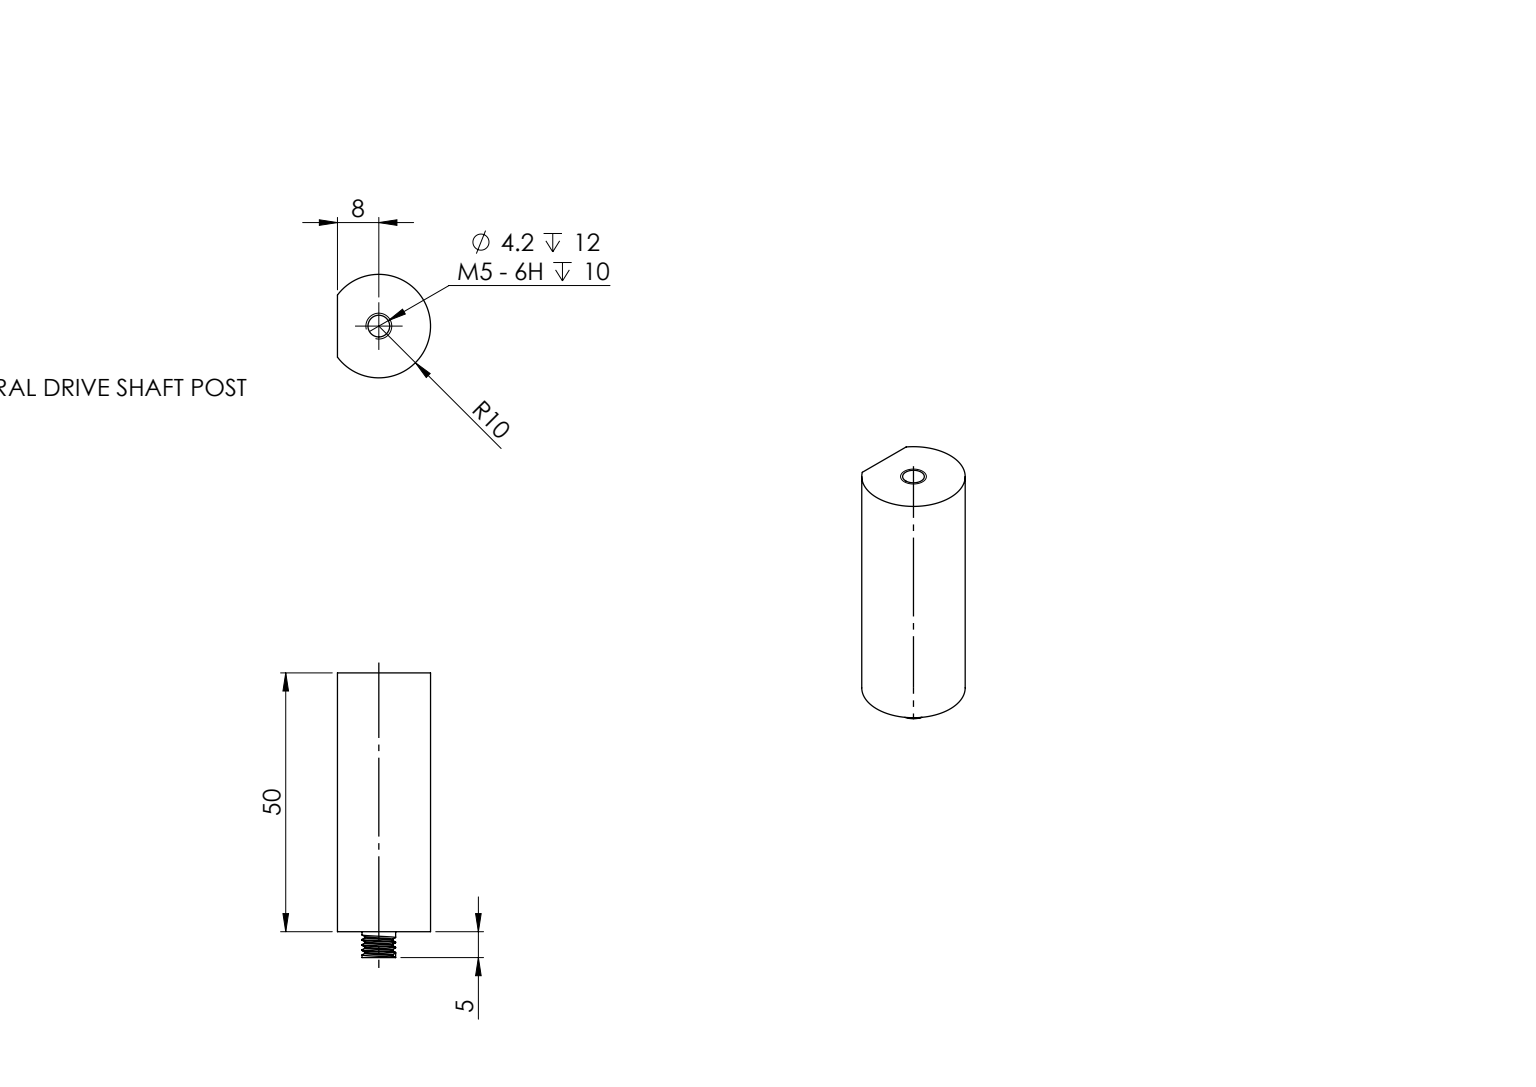
ISO-10303-21;
HEADER;
FILE_DESCRIPTION (('STEP AP214'),
    '1' );
FILE_NAME ('Central Drive Shaft Post.step',
    '2026-10-08T14:59:03',
    ( '' ),
    ( '' ),
    'SwSTEP 2.0',
    'SolidWorks 2026',
    '' );
FILE_SCHEMA (( 'AUTOMOTIVE_DESIGN' ));
ENDSEC;

DATA;
#13=CARTESIAN_POINT ( 'NONE',  ( -2.298097038856279806, 112.6250000000000000, -2.298097038856279362 ) ) ;
#14=CARTESIAN_POINT ( 'NONE',  ( 1.658621287961228320E-16, 111.8124999986344079, 2.708734124999999882 ) ) ;
#16=AXIS2_PLACEMENT_3D ( 'NONE', #8718, #1999, #3870 ) ;
#26=CARTESIAN_POINT ( 'NONE',  ( 0.000000000000000000, 153.0000000000000000, 2.099999999999998312 ) ) ;
#35=CARTESIAN_POINT ( 'NONE',  ( 3.250000000000000444, 113.0625000000000000, 1.346194077712559167 ) ) ;
#42=ORIENTED_EDGE ( 'NONE', *, *, #4224, .F. ) ;
#57=CARTESIAN_POINT ( 'NONE',  ( -1.915364268218909150, 112.6874999986344079, 1.915364268218909594 ) ) ;
#60=ORIENTED_EDGE ( 'NONE', *, *, #4267, .T. ) ;
#74=CARTESIAN_POINT ( 'NONE',  ( -3.250000000000000444, 111.5000000000000000, 3.980102097228898231E-16 ) ) ;
#90=ORIENTED_EDGE ( 'NONE', *, *, #4166, .T. ) ;
#101=CARTESIAN_POINT ( 'NONE',  ( -2.298097038856279362, 111.3750000000000000, 2.298097038856279806 ) ) ;
#103=CARTESIAN_POINT ( 'NONE',  ( 1.121994411437818862, 110.4999999986344079, 2.708734125000000326 ) ) ;
#122=CARTESIAN_POINT ( 'NONE',  ( -1.121994411437818862, 113.6249999986344079, 2.708734125000000326 ) ) ;
#124=EDGE_CURVE ( 'NONE', #2418, #8492, #10933, .T. ) ;
#126=EDGE_LOOP ( 'NONE', ( #8083, #10579, #5308 ) ) ;
#133=CARTESIAN_POINT ( 'NONE',  ( -1.346194077712560944, 110.3125000000000000, 3.249999999999998668 ) ) ;
#136=CARTESIAN_POINT ( 'NONE',  ( 1.915364268218908705, 114.4374999986344079, -1.915364268218909594 ) ) ;
#138=CARTESIAN_POINT ( 'NONE',  ( 1.915364268218909150, 112.6874999986344079, 1.915364268218909150 ) ) ;
#148=ADVANCED_FACE ( 'NONE', ( #9407 ), #4682, .T. ) ;
#153=EDGE_CURVE ( 'NONE', #12150, #6802, #1695, .T. ) ;
#167=CARTESIAN_POINT ( 'NONE',  ( 1.658621287961228566E-16, 110.5624999986344079, 2.708734125000000326 ) ) ;
#183=CARTESIAN_POINT ( 'NONE',  ( -2.708734125000000326, 113.7499999986343937, 1.121994411437818862 ) ) ;
#184=CARTESIAN_POINT ( 'NONE',  ( -5.970153145843347347E-16, 113.6249999972688158, -3.250000000000000444 ) ) ;
#196=EDGE_CURVE ( 'NONE', #8201, #12241, #11240, .T. ) ;
#217=AXIS2_PLACEMENT_3D ( 'NONE', #5378, #8352, #3567 ) ;
#232=CARTESIAN_POINT ( 'NONE',  ( 2.708734125000000326, 110.3749999986344221, 1.121994411437818862 ) ) ;
#239=CARTESIAN_POINT ( 'NONE',  ( -3.250000000000000444, 111.3124999972687874, 1.346194077712559167 ) ) ;
#245=ORIENTED_EDGE ( 'NONE', *, *, #2310, .T. ) ;
#246=CARTESIAN_POINT ( 'NONE',  ( -2.708734125000000326, 110.7499999986343937, 1.121994411437818862 ) ) ;
#249=EDGE_CURVE ( 'NONE', #1174, #5753, #3010, .T. ) ;
#263=CARTESIAN_POINT ( 'NONE',  ( -1.915364268218909594, 114.1874999986344079, -1.915364268218908927 ) ) ;
#265=CARTESIAN_POINT ( 'NONE',  ( -1.915364268218909594, 113.1874999986344079, -1.915364268218908927 ) ) ;
#289=CARTESIAN_POINT ( 'NONE',  ( -1.121994411437820416, 110.9999999986343937, -2.708734124999999882 ) ) ;
#291=CARTESIAN_POINT ( 'NONE',  ( 1.990051048614449116E-16, 113.1249999972688158, 3.250000000000000444 ) ) ;
#292=( GEOMETRIC_REPRESENTATION_CONTEXT ( 3 ) GLOBAL_UNCERTAINTY_ASSIGNED_CONTEXT ( ( #10000 ) ) GLOBAL_UNIT_ASSIGNED_CONTEXT ( ( #7020, #9690, #6089 ) ) REPRESENTATION_CONTEXT ( 'NONE', 'WORKASPACE' ) );
#307=CLOSED_SHELL ( 'NONE', ( #11275, #6512, #7917, #11356, #3953, #6283, #1808, #1279, #6245, #3383, #11433, #6682, #11026, #12101, #4967, #2002, #12145, #10844, #5599, #3792, #148, #6574, #11472, #11341, #11642, #320 ) ) ;
#308=CARTESIAN_POINT ( 'NONE',  ( -4.975863863883684959E-16, 111.0624999986344079, -2.708734125000000326 ) ) ;
#310=CARTESIAN_POINT ( 'NONE',  ( -2.298097038856279362, 114.2499999972688158, 2.298097038856279806 ) ) ;
#320=ADVANCED_FACE ( 'NONE', ( #4060 ), #2414, .F. ) ;
#324=ORIENTED_EDGE ( 'NONE', *, *, #11720, .F. ) ;
#325=CARTESIAN_POINT ( 'NONE',  ( -8.000000000000000000, 115.0000000000000000, 5.999999999999998224 ) ) ;
#337=VECTOR ( 'NONE', #4948, 1000.000000000000227 ) ;
#340=CARTESIAN_POINT ( 'NONE',  ( 1.121994411437819084, 110.4999999986343937, 2.708734125000000326 ) ) ;
#341=ORIENTED_EDGE ( 'NONE', *, *, #9592, .T. ) ;
#348=EDGE_CURVE ( 'NONE', #9835, #9973, #11157, .T. ) ;
#350=CARTESIAN_POINT ( 'NONE',  ( 2.708734124999999882, 114.2499999986344079, -1.121994411437820638 ) ) ;
#359=ORIENTED_EDGE ( 'NONE', *, *, #2691, .F. ) ;
#360=CARTESIAN_POINT ( 'NONE',  ( 0.000000000000000000, 165.0000000000000000, 0.000000000000000000 ) ) ;
#363=CARTESIAN_POINT ( 'NONE',  ( 0.000000000000000000, 165.0000000000000000, 0.000000000000000000 ) ) ;
#398=CARTESIAN_POINT ( 'NONE',  ( -3.250000000000000444, 112.3124999972687874, 1.346194077712559167 ) ) ;
#403=ORIENTED_EDGE ( 'NONE', *, *, #1223, .T. ) ;
#416=CARTESIAN_POINT ( 'NONE',  ( -2.708734125000000326, 113.8124999986344079, 3.317242575922457132E-16 ) ) ;
#418=FACE_OUTER_BOUND ( 'NONE', #10833, .T. ) ;
#421=VERTEX_POINT ( 'NONE', #5825 ) ;
#438=ORIENTED_EDGE ( 'NONE', *, *, #2215, .F. ) ;
#454=CARTESIAN_POINT ( 'NONE',  ( 3.250000000000000444, 111.0000000000000000, 0.000000000000000000 ) ) ;
#478=CARTESIAN_POINT ( 'NONE',  ( -4.975863863883684959E-16, 114.0624999986344079, -2.708734125000000326 ) ) ;
#480=CYLINDRICAL_SURFACE ( 'NONE', #7570, 3.250000000000000444 ) ;
#489=CARTESIAN_POINT ( 'NONE',  ( 2.298097038856279806, 113.9999999972688158, 2.298097038856279806 ) ) ;
#494=ORIENTED_EDGE ( 'NONE', *, *, #4807, .F. ) ;
#499=CARTESIAN_POINT ( 'NONE',  ( 1.990051048614449116E-16, 114.1249999972688158, 3.250000000000000444 ) ) ;
#509=CARTESIAN_POINT ( 'NONE',  ( 2.298097038856279806, 112.1250000000000000, 2.298097038856279806 ) ) ;
#525=CARTESIAN_POINT ( 'NONE',  ( 2.708734124999999882, 112.2499999986343937, -1.121994411437820416 ) ) ;
#529=ORIENTED_EDGE ( 'NONE', *, *, #10124, .T. ) ;
#540=CARTESIAN_POINT ( 'NONE',  ( 1.121994411437819528, 114.1249999986344079, -2.708734124999999882 ) ) ;
#541=CARTESIAN_POINT ( 'NONE',  ( -1.121994411437819084, 110.8749999986343937, 2.708734124999999882 ) ) ;
#551=ORIENTED_EDGE ( 'NONE', *, *, #4637, .F. ) ;
#586=CARTESIAN_POINT ( 'NONE',  ( 1.915364268218908927, 113.1874999986344079, -1.915364268218909816 ) ) ;
#589=MANIFOLD_SOLID_BREP ( 'Thread1', #307 ) ;
#605=CARTESIAN_POINT ( 'NONE',  ( 1.346194077712559389, 113.1875000000000142, 3.250000000000000444 ) ) ;
#618=EDGE_LOOP ( 'NONE', ( #8709, #551, #5002, #341 ) ) ;
#622=DIRECTION ( 'NONE',  ( -0.000000000000000000, 1.000000000000000000, -0.000000000000000000 ) ) ;
#627=CARTESIAN_POINT ( 'NONE',  ( -3.250000000000000444, 114.3749999972688158, 3.980102097228898231E-16 ) ) ;
#637=CARTESIAN_POINT ( 'NONE',  ( 2.298097038856278918, 111.8750000000000000, -2.298097038856279806 ) ) ;
#653=CARTESIAN_POINT ( 'NONE',  ( 1.121994411437819528, 114.1249999986344079, -2.708734124999999882 ) ) ;
#655=CARTESIAN_POINT ( 'NONE',  ( 1.121994411437818862, 111.7499999986344079, 2.708734124999999882 ) ) ;
#663=LINE ( 'NONE', #3470, #9246 ) ;
#665=DIRECTION ( 'NONE',  ( -0.000000000000000000, -1.000000000000000000, -0.000000000000000000 ) ) ;
#668=CARTESIAN_POINT ( 'NONE',  ( -5.970153145843347347E-16, 112.7500000000000000, -3.250000000000000444 ) ) ;
#685=AXIS2_PLACEMENT_3D ( 'NONE', #9077, #3726, #10139 ) ;
#704=CARTESIAN_POINT ( 'NONE',  ( 0.000000000000000000, 110.0000000000000000, 0.000000000000000000 ) ) ;
#705=MECHANICAL_DESIGN_GEOMETRIC_PRESENTATION_REPRESENTATION('',(#6077),#292);
#707=VECTOR ( 'NONE', #7770, 1000.000000000000000 ) ;
#709=EDGE_LOOP ( 'NONE', ( #12315, #3463 ) ) ;
#723=CARTESIAN_POINT ( 'NONE',  ( -2.708734124999999882, 110.9999999986343937, 1.121994411437818862 ) ) ;
#725=AXIS2_PLACEMENT_3D ( 'NONE', #3282, #2404, #5224 ) ;
#738=CARTESIAN_POINT ( 'NONE',  ( 3.250000000000000444, 113.0000000000000000, 0.000000000000000000 ) ) ;
#769=CARTESIAN_POINT ( 'NONE',  ( 2.708734124999999437, 114.4999999986344079, -1.121994411437820638 ) ) ;
#772=ORIENTED_EDGE ( 'NONE', *, *, #7001, .F. ) ;
#782=ORIENTED_EDGE ( 'NONE', *, *, #11976, .F. ) ;
#785=CARTESIAN_POINT ( 'NONE',  ( 1.915364268218908705, 113.4374999986344079, -1.915364268218909594 ) ) ;
#796=CARTESIAN_POINT ( 'NONE',  ( 2.298097038856279806, 112.1250000000000000, 2.298097038856279806 ) ) ;
#804=LINE ( 'NONE', #2726, #2890 ) ;
#829=CARTESIAN_POINT ( 'NONE',  ( 2.708734124999999882, 114.5624999986344079, 0.000000000000000000 ) ) ;
#843=CARTESIAN_POINT ( 'NONE',  ( -4.975863863883684959E-16, 113.3124999986344079, -2.708734124999999882 ) ) ;
#850=AXIS2_PLACEMENT_3D ( 'NONE', #3146, #7011, #2387 ) ;
#859=CARTESIAN_POINT ( 'NONE',  ( 2.298097038856278918, 112.7499999972688158, -2.298097038856279806 ) ) ;
#861=VERTEX_POINT ( 'NONE', #10306 ) ;
#887=CARTESIAN_POINT ( 'NONE',  ( 1.121994411437818862, 112.7499999986343937, 2.708734124999999882 ) ) ;
#889=CARTESIAN_POINT ( 'NONE',  ( 2.298097038856278918, 113.8750000000000000, -2.298097038856279806 ) ) ;
#902=CARTESIAN_POINT ( 'NONE',  ( 2.708734124999999882, 111.5624999986344079, 0.000000000000000000 ) ) ;
#917=CARTESIAN_POINT ( 'NONE',  ( -5.970153145843347347E-16, 112.7500000000000000, -3.250000000000000444 ) ) ;
#947=DIRECTION ( 'NONE',  ( 0.000000000000000000, 0.000000000000000000, -1.000000000000000000 ) ) ;
#951=CARTESIAN_POINT ( 'NONE',  ( 2.708734124999999882, 112.5624999986344079, 0.000000000000000000 ) ) ;
#952=CARTESIAN_POINT ( 'NONE',  ( -2.298097038856279362, 111.2499999972688158, 2.298097038856279806 ) ) ;
#965=CARTESIAN_POINT ( 'NONE',  ( -2.708734124999999882, 114.0624999986344079, 3.317242575922456639E-16 ) ) ;
#977=LINE ( 'NONE', #3904, #10328 ) ;
#995=CARTESIAN_POINT ( 'NONE',  ( -3.250000000000000444, 113.3124999972687874, 1.346194077712559167 ) ) ;
#1010=CARTESIAN_POINT ( 'NONE',  ( -2.708734125000000326, 113.1249999986343937, -1.121994411437818195 ) ) ;
#1011=CARTESIAN_POINT ( 'NONE',  ( -3.250000000000000444, 112.3749999972688158, 3.980102097228898231E-16 ) ) ;
#1025=DIRECTION ( 'NONE',  ( 0.000000000000000000, 0.000000000000000000, 1.000000000000000000 ) ) ;
#1026=CARTESIAN_POINT ( 'NONE',  ( -3.250000000000001776, 113.5625000000000000, -1.346194077712558723 ) ) ;
#1039=( LENGTH_UNIT ( ) NAMED_UNIT ( * ) SI_UNIT ( .MILLI., .METRE. ) );
#1041=APPLICATION_CONTEXT ( 'automotive_design' ) ;
#1053=CARTESIAN_POINT ( 'NONE',  ( -2.298097038856279362, 113.2499999972688158, 2.298097038856279806 ) ) ;
#1056=LINE ( 'NONE', #1122, #1359 ) ;
#1068=CARTESIAN_POINT ( 'NONE',  ( 1.915364268218908927, 113.1874999986344079, -1.915364268218909816 ) ) ;
#1070=CARTESIAN_POINT ( 'NONE',  ( -3.250000000000001776, 113.4374999972688300, -1.346194077712558723 ) ) ;
#1076=CARTESIAN_POINT ( 'NONE',  ( 0.000000000000000000, 165.0000000000000000, 0.000000000000000000 ) ) ;
#1099=CARTESIAN_POINT ( 'NONE',  ( -1.915364268218909150, 110.6874999986344079, 1.915364268218909594 ) ) ;
#1115=CARTESIAN_POINT ( 'NONE',  ( -2.708734125000000326, 110.8124999986344079, 3.317242575922457132E-16 ) ) ;
#1122=CARTESIAN_POINT ( 'NONE',  ( 2.571758278209433575E-16, 165.0000000000000000, -2.099999999999993427 ) ) ;
#1133=CARTESIAN_POINT ( 'NONE',  ( -1.915364268218909816, 113.9374999986344079, -1.915364268218909150 ) ) ;
#1134=CARTESIAN_POINT ( 'NONE',  ( -1.346194077712560944, 112.5624999972688158, -3.249999999999999556 ) ) ;
#1149=PLANE ( 'NONE',  #1794 ) ;
#1152=EDGE_CURVE ( 'NONE', #5494, #3256, #5047, .T. ) ;
#1153=VERTEX_POINT ( 'NONE', #9045 ) ;
#1160=CARTESIAN_POINT ( 'NONE',  ( 2.708734125000000326, 111.3124999986344079, 0.000000000000000000 ) ) ;
#1168=CARTESIAN_POINT ( 'NONE',  ( -2.708734125000000326, 112.1249999986343937, -1.121994411437818195 ) ) ;
#1174=VERTEX_POINT ( 'NONE', #4317 ) ;
#1185=ORIENTED_EDGE ( 'NONE', *, *, #4989, .T. ) ;
#1189=PRODUCT_CONTEXT ( 'NONE', #1041, 'mechanical' ) ;
#1194=CARTESIAN_POINT ( 'NONE',  ( 2.708734125000000326, 111.3124999986344079, 0.000000000000000000 ) ) ;
#1195=CARTESIAN_POINT ( 'NONE',  ( -3.250000000000000444, 111.3749999972688158, 3.980102097228898231E-16 ) ) ;
#1210=CARTESIAN_POINT ( 'NONE',  ( 1.121994411437819084, 112.3749999986344079, -2.708734124999999437 ) ) ;
#1223=EDGE_CURVE ( 'NONE', #9534, #3450, #11896, .T. ) ;
#1229=CARTESIAN_POINT ( 'NONE',  ( 3.980102097228898231E-16, 110.0000000000000000, -3.250000000000000444 ) ) ;
#1235=CARTESIAN_POINT ( 'NONE',  ( 2.708734125000000326, 112.3749999986344221, 1.121994411437818862 ) ) ;
#1239=( BOUNDED_CURVE ( )  B_SPLINE_CURVE ( 2, ( #499, #8154, #2434, #10086, #627, #11860, #10030, #5367, #11982 ),
 .UNSPECIFIED., .F., .F. ) 
 B_SPLINE_CURVE_WITH_KNOTS ( ( 3, 2, 2, 2, 3 ),
 ( 0.8125000000000006661, 0.8437500000000006661, 0.8750000000000006661, 0.9062500000000007772, 0.9375000000000007772 ),
 .UNSPECIFIED. ) 
 CURVE ( )  GEOMETRIC_REPRESENTATION_ITEM ( )  RATIONAL_B_SPLINE_CURVE ( ( 0.9999999999999983347, 0.9238795325112884038, 1.000000000000000000, 0.9238795325112867385, 1.000000000000000000, 0.9238795325112867385, 1.000000000000000000, 0.9238795325112848511, 1.000000000000001998 ) ) 
 REPRESENTATION_ITEM ( '' )  );
#1252=CARTESIAN_POINT ( 'NONE',  ( 2.708734124999999882, 111.2499999986344079, -1.121994411437820638 ) ) ;
#1253=CARTESIAN_POINT ( 'NONE',  ( 3.249999999999999556, 113.8124999972688016, -1.346194077712561610 ) ) ;
#1256=EDGE_CURVE ( 'NONE', #1921, #9884, #2097, .T. ) ;
#1263=CARTESIAN_POINT ( 'NONE',  ( -2.298097038856279362, 110.3750000000000000, 2.298097038856279806 ) ) ;
#1267=ORIENTED_EDGE ( 'NONE', *, *, #6550, .T. ) ;
#1274=ORIENTED_EDGE ( 'NONE', *, *, #3107, .T. ) ;
#1277=CARTESIAN_POINT ( 'NONE',  ( 1.990051048614449116E-16, 110.2500000000000000, 3.250000000000000444 ) ) ;
#1279=ADVANCED_FACE ( 'NONE', ( #5699 ), #5517, .T. ) ;
#1295=CARTESIAN_POINT ( 'NONE',  ( -1.915364268218909150, 111.6874999986344079, 1.915364268218909594 ) ) ;
#1314=CARTESIAN_POINT ( 'NONE',  ( -1.915364268218909150, 111.6874999986344079, 1.915364268218909594 ) ) ;
#1323=CARTESIAN_POINT ( 'NONE',  ( 0.000000000000000000, 110.0000000000000000, 0.000000000000000000 ) ) ;
#1347=SURFACE_SIDE_STYLE ('',( #4211 ) ) ;
#1355=CARTESIAN_POINT ( 'NONE',  ( -2.708734125000000326, 111.7499999986344079, 1.121994411437818862 ) ) ;
#1357=CARTESIAN_POINT ( 'NONE',  ( 0.000000000000000000, 165.0000000000000000, 0.000000000000000000 ) ) ;
#1359=VECTOR ( 'NONE', #1537, 1000.000000000000000 ) ;
#1377=EDGE_CURVE ( 'NONE', #8030, #8106, #3017, .T. ) ;
#1395=CARTESIAN_POINT ( 'NONE',  ( 3.249999999999999556, 110.9375000000000000, -1.346194077712561166 ) ) ;
#1417=CARTESIAN_POINT ( 'NONE',  ( 0.000000000000000000, 165.0000000000000000, -9.999999999999998224 ) ) ;
#1419=CARTESIAN_POINT ( 'NONE',  ( -1.915364268218909150, 113.6874999986344079, 1.915364268218909594 ) ) ;
#1459=CARTESIAN_POINT ( 'NONE',  ( 1.990051048614449116E-16, 111.2500000000000000, 3.250000000000000444 ) ) ;
#1462=ORIENTED_EDGE ( 'NONE', *, *, #11573, .T. ) ;
#1463=CARTESIAN_POINT ( 'NONE',  ( 1.990051048614449116E-16, 113.1249999972688158, 3.250000000000000444 ) ) ;
#1466=CARTESIAN_POINT ( 'NONE',  ( -1.915364268218909150, 112.6874999986344079, 1.915364268218909594 ) ) ;
#1476=DIRECTION ( 'NONE',  ( 0.000000000000000000, 0.000000000000000000, 1.000000000000000000 ) ) ;
#1481=CARTESIAN_POINT ( 'NONE',  ( 2.708734124999999882, 113.2499999986344079, -1.121994411437820638 ) ) ;
#1497=AXIS2_PLACEMENT_3D ( 'NONE', #7319, #7066, #11118 ) ;
#1502=PLANE ( 'NONE',  #9393 ) ;
#1520=DIRECTION ( 'NONE',  ( 0.000000000000000000, 0.000000000000000000, 1.000000000000000000 ) ) ;
#1528=CARTESIAN_POINT ( 'NONE',  ( -1.915364268218909816, 111.9374999986344079, -1.915364268218909150 ) ) ;
#1532=( LENGTH_UNIT ( ) NAMED_UNIT ( * ) SI_UNIT ( .MILLI., .METRE. ) );
#1534=UNCERTAINTY_MEASURE_WITH_UNIT (LENGTH_MEASURE( 1.000000000000000082E-05 ), #1039, 'distance_accuracy_value', 'NONE');
#1537=DIRECTION ( 'NONE',  ( -0.000000000000000000, 1.000000000000000000, -0.000000000000000000 ) ) ;
#1544=CARTESIAN_POINT ( 'NONE',  ( -2.298097038856279362, 112.3750000000000000, 2.298097038856279806 ) ) ;
#1545=CARTESIAN_POINT ( 'NONE',  ( 2.708734124999999882, 110.6249999986343937, 1.121994411437819084 ) ) ;
#1547=CARTESIAN_POINT ( 'NONE',  ( 3.249999999999999556, 112.8124999972687874, -1.346194077712561166 ) ) ;
#1550=VERTEX_POINT ( 'NONE', #9028 ) ;
#1561=VECTOR ( 'NONE', #11409, 1000.000000000000000 ) ;
#1568=AXIS2_PLACEMENT_3D ( 'NONE', #1776, #5529, #7332 ) ;
#1575=CARTESIAN_POINT ( 'NONE',  ( -5.970153145843347347E-16, 111.7500000000000000, -3.250000000000000444 ) ) ;
#1587=CARTESIAN_POINT ( 'NONE',  ( 1.915364268218909594, 112.4374999986344079, 1.915364268218909594 ) ) ;
#1590=CARTESIAN_POINT ( 'NONE',  ( -2.708734124999999882, 112.0624999986344079, 3.317242575922456639E-16 ) ) ;
#1603=CARTESIAN_POINT ( 'NONE',  ( 2.298097038856278918, 111.7499999972688158, -2.298097038856279806 ) ) ;
#1604=CARTESIAN_POINT ( 'NONE',  ( -2.298097038856279806, 111.6250000000000000, -2.298097038856279362 ) ) ;
#1612=AXIS2_PLACEMENT_3D ( 'NONE', #9562, #7823, #5032 ) ;
#1627=FACE_OUTER_BOUND ( 'NONE', #4261, .T. ) ;
#1640=EDGE_LOOP ( 'NONE', ( #4892, #782, #4872, #2457 ) ) ;
#1641=CARTESIAN_POINT ( 'NONE',  ( 2.708734124999999882, 110.5624999986344079, 0.000000000000000000 ) ) ;
#1652=CARTESIAN_POINT ( 'NONE',  ( -1.121994411437820194, 111.2499999986344079, -2.708734124999999437 ) ) ;
#1664=CARTESIAN_POINT ( 'NONE',  ( 1.346194077712559833, 112.8124999999999858, -3.250000000000000000 ) ) ;
#1676=EDGE_LOOP ( 'NONE', ( #6465, #3810, #10461, #7615 ) ) ;
#1686=DIRECTION ( 'NONE',  ( -0.000000000000000000, 1.000000000000000000, -0.000000000000000000 ) ) ;
#1695=( BOUNDED_CURVE ( )  B_SPLINE_CURVE ( 2, ( #2630, #1701, #889, #7437, #8474 ),
 .UNSPECIFIED., .F., .F. ) 
 B_SPLINE_CURVE_WITH_KNOTS ( ( 3, 2, 3 ),
 ( 0.9375000000000007772, 0.9687500000000004441, 1.000000000000000000 ),
 .UNSPECIFIED. ) 
 CURVE ( )  GEOMETRIC_REPRESENTATION_ITEM ( )  RATIONAL_B_SPLINE_CURVE ( ( 0.9999999999999981126, 0.9238795325112886259, 1.000000000000000000, 0.9238795325112867385, 1.000000000000000000 ) ) 
 REPRESENTATION_ITEM ( '' )  );
#1700=CARTESIAN_POINT ( 'NONE',  ( -1.121994411437818862, 112.8749999986344079, 2.708734124999999882 ) ) ;
#1701=CARTESIAN_POINT ( 'NONE',  ( 1.346194077712585591, 113.8125000000000142, -3.249999999999974687 ) ) ;
#1704=ORIENTED_EDGE ( 'NONE', *, *, #10723, .F. ) ;
#1715=CARTESIAN_POINT ( 'NONE',  ( -2.708734124999999882, 113.0624999986344079, 3.317242575922456639E-16 ) ) ;
#1722=CYLINDRICAL_SURFACE ( 'NONE', #1568, 3.250000000000000444 ) ;
#1730=CARTESIAN_POINT ( 'NONE',  ( -3.250000000000001776, 111.5624999999999858, -1.346194077712558723 ) ) ;
#1733=CARTESIAN_POINT ( 'NONE',  ( 1.990051048614449116E-16, 113.1249999972688158, 3.250000000000000444 ) ) ;
#1754=LINE ( 'NONE', #5438, #2930 ) ;
#1758=CARTESIAN_POINT ( 'NONE',  ( 1.658621287961228320E-16, 113.8124999986344079, 2.708734124999999882 ) ) ;
#1764=ORIENTED_EDGE ( 'NONE', *, *, #124, .F. ) ;
#1770=CARTESIAN_POINT ( 'NONE',  ( 1.658621287961228320E-16, 111.8124999986344079, 2.708734124999999882 ) ) ;
#1771=CARTESIAN_POINT ( 'NONE',  ( -1.121994411437820194, 111.2499999986344079, -2.708734124999999437 ) ) ;
#1776=CARTESIAN_POINT ( 'NONE',  ( 0.000000000000000000, 110.0000000000000000, 0.000000000000000000 ) ) ;
#1794=AXIS2_PLACEMENT_3D ( 'NONE', #6754, #11627, #4951 ) ;
#1806=LINE ( 'NONE', #11225, #8415 ) ;
#1808=ADVANCED_FACE ( 'NONE', ( #2163 ), #10942, .T. ) ;
#1813=CARTESIAN_POINT ( 'NONE',  ( 3.250000000000000444, 110.0000000000000000, 0.000000000000000000 ) ) ;
#1814=VECTOR ( 'NONE', #6503, 1000.000000000000000 ) ;
#1817=CARTESIAN_POINT ( 'NONE',  ( -4.975863863883684959E-16, 112.3124999986344079, -2.708734124999999882 ) ) ;
#1826=CARTESIAN_POINT ( 'NONE',  ( 3.250000000000000444, 110.0624999999999858, 1.346194077712559167 ) ) ;
#1832=CARTESIAN_POINT ( 'NONE',  ( 1.915364268218909150, 110.6874999986344079, 1.915364268218909150 ) ) ;
#1874=CARTESIAN_POINT ( 'NONE',  ( 1.915364268218908705, 114.4374999986344079, -1.915364268218909594 ) ) ;
#1876=CARTESIAN_POINT ( 'NONE',  ( -2.298097038856279806, 111.4999999972688158, -2.298097038856279362 ) ) ;
#1883=CARTESIAN_POINT ( 'NONE',  ( -5.970153145843347347E-16, 112.7500000000000000, -3.250000000000000444 ) ) ;
#1921=VERTEX_POINT ( 'NONE', #11007 ) ;
#1927=ORIENTED_EDGE ( 'NONE', *, *, #4103, .F. ) ;
#1933=CARTESIAN_POINT ( 'NONE',  ( -5.970153145843347347E-16, 111.6249999972688158, -3.250000000000000444 ) ) ;
#1942=CARTESIAN_POINT ( 'NONE',  ( 1.658621287961228320E-16, 112.8124999986344079, 2.708734124999999882 ) ) ;
#1943=CARTESIAN_POINT ( 'NONE',  ( 1.346194077712559389, 111.0624999972688016, 3.250000000000000444 ) ) ;
#1948=CARTESIAN_POINT ( 'NONE',  ( 2.298097038856279806, 110.1250000000000000, 2.298097038856279806 ) ) ;
#1953=CARTESIAN_POINT ( 'NONE',  ( -1.121994411437820194, 114.2499999986344079, -2.708734124999999437 ) ) ;
#1954=CARTESIAN_POINT ( 'NONE',  ( 2.298097038856278918, 113.8750000000000000, -2.298097038856279806 ) ) ;
#1959=MECHANICAL_DESIGN_GEOMETRIC_PRESENTATION_REPRESENTATION('',(#10160),#3359);
#1999=DIRECTION ( 'NONE',  ( 0.000000000000000000, 1.000000000000000000, 0.000000000000000000 ) ) ;
#2001=CARTESIAN_POINT ( 'NONE',  ( -2.708734125000000326, 112.8124999986344079, 3.317242575922457132E-16 ) ) ;
#2002=ADVANCED_FACE ( 'NONE', ( #3469 ), #11075, .F. ) ;
#2003=CARTESIAN_POINT ( 'NONE',  ( 2.298097038856278918, 111.7499999972688158, -2.298097038856279806 ) ) ;
#2018=CARTESIAN_POINT ( 'NONE',  ( 0.000000000000000000, 165.0000000000000000, 0.000000000000000000 ) ) ;
#2021=CARTESIAN_POINT ( 'NONE',  ( 1.915364268218909150, 113.6874999986344079, 1.915364268218909150 ) ) ;
#2029=AXIS2_PLACEMENT_3D ( 'NONE', #4331, #8256, #6334 ) ;
#2034=CARTESIAN_POINT ( 'NONE',  ( -1.915364268218909816, 110.9374999986344079, -1.915364268218909150 ) ) ;
#2066=CARTESIAN_POINT ( 'NONE',  ( 1.346194077712559833, 112.6874999972688158, -3.250000000000000000 ) ) ;
#2079=CARTESIAN_POINT ( 'NONE',  ( 1.121994411437819084, 114.3749999986344221, -2.708734124999999437 ) ) ;
#2081=CARTESIAN_POINT ( 'NONE',  ( 2.708734124999999437, 114.4999999986344079, -1.121994411437820416 ) ) ;
#2093=CARTESIAN_POINT ( 'NONE',  ( -2.708734125000000326, 110.7499999986343937, 1.121994411437819084 ) ) ;
#2097=( BOUNDED_CURVE ( )  B_SPLINE_CURVE ( 2, ( #8481, #11182, #3753, #2636, #2697, #6444, #6509, #10235, #1883 ),
 .UNSPECIFIED., .F., .F. ) 
 B_SPLINE_CURVE_WITH_KNOTS ( ( 3, 2, 2, 2, 3 ),
 ( 0.5625000000000004441, 0.5937500000000004441, 0.6250000000000004441, 0.6562500000000005551, 0.6875000000000005551 ),
 .UNSPECIFIED. ) 
 CURVE ( )  GEOMETRIC_REPRESENTATION_ITEM ( )  RATIONAL_B_SPLINE_CURVE ( ( 0.9999999999999988898, 0.9238795325112878487, 1.000000000000000000, 0.9238795325112867385, 1.000000000000000000, 0.9238795325112867385, 1.000000000000000000, 0.9238795325112854062, 1.000000000000001332 ) ) 
 REPRESENTATION_ITEM ( '' )  );
#2103=FILL_AREA_STYLE ('',( #3219 ) ) ;
#2109=CARTESIAN_POINT ( 'NONE',  ( 1.990051048614449116E-16, 111.2500000000000000, 3.250000000000000444 ) ) ;
#2116=ORIENTED_EDGE ( 'NONE', *, *, #4989, .F. ) ;
#2125=FACE_BOUND ( 'NONE', #709, .T. ) ;
#2127=CARTESIAN_POINT ( 'NONE',  ( -1.915364268218909816, 111.9374999986344079, -1.915364268218909150 ) ) ;
#2128=CARTESIAN_POINT ( 'NONE',  ( -1.346194077712559389, 113.1874999972688016, 3.250000000000000444 ) ) ;
#2141=CARTESIAN_POINT ( 'NONE',  ( 0.000000000000000000, 153.0000000000000000, 0.000000000000000000 ) ) ;
#2143=CARTESIAN_POINT ( 'NONE',  ( 2.708734124999999437, 112.4999999986343937, -1.121994411437820416 ) ) ;
#2150=DIRECTION ( 'NONE',  ( 0.000000000000000000, 0.000000000000000000, 1.000000000000000000 ) ) ;
#2163=FACE_OUTER_BOUND ( 'NONE', #8054, .T. ) ;
#2179=CARTESIAN_POINT ( 'NONE',  ( -1.121994411437818862, 111.6249999986344079, 2.708734125000000326 ) ) ;
#2180=CARTESIAN_POINT ( 'NONE',  ( 1.990051048614449116E-16, 114.1249999972688158, 3.250000000000000444 ) ) ;
#2198=CARTESIAN_POINT ( 'NONE',  ( 2.708734124999999882, 111.6249999986343937, 1.121994411437819084 ) ) ;
#2209=CARTESIAN_POINT ( 'NONE',  ( 0.000000000000000000, 115.0000000000000000, -9.999999999999998224 ) ) ;
#2211=DIRECTION ( 'NONE',  ( 0.000000000000000000, 0.000000000000000000, -1.000000000000000000 ) ) ;
#2215=EDGE_CURVE ( 'NONE', #9788, #5829, #977, .T. ) ;
#2217=SURFACE_STYLE_USAGE ( .BOTH. , #1347 ) ;
#2220=SURFACE_SIDE_STYLE ('',( #11703 ) ) ;
#2221=AXIS2_PLACEMENT_3D ( 'NONE', #4678, #8469, #12295 ) ;
#2227=CARTESIAN_POINT ( 'NONE',  ( -4.975863863883684959E-16, 113.0624999986344079, -2.708734125000000326 ) ) ;
#2231=ORIENTED_EDGE ( 'NONE', *, *, #6662, .T. ) ;
#2241=CARTESIAN_POINT ( 'NONE',  ( -2.708734125000000770, 110.8749999986343937, -1.121994411437818639 ) ) ;
#2248=DIRECTION ( 'NONE',  ( -0.000000000000000000, 1.000000000000000000, -0.000000000000000000 ) ) ;
#2260=CARTESIAN_POINT ( 'NONE',  ( 1.990051048614449116E-16, 112.1249999972688158, 3.250000000000000444 ) ) ;
#2268=EDGE_LOOP ( 'NONE', ( #10266, #8033, #7306, #7027, #11755, #11420, #6855, #438 ) ) ;
#2271=CARTESIAN_POINT ( 'NONE',  ( 0.000000000000000000, 110.0000000000000000, 0.000000000000000000 ) ) ;
#2276=SHAPE_REPRESENTATION_RELATIONSHIP ( 'NONE' , 'NONE' ,  #7136, #7202 ) ;
#2278=ORIENTED_EDGE ( 'NONE', *, *, #9929, .T. ) ;
#2288=CARTESIAN_POINT ( 'NONE',  ( -3.250000000000000444, 110.4375000000000000, 1.346194077712559389 ) ) ;
#2310=EDGE_CURVE ( 'NONE', #2754, #4316, #4490, .T. ) ;
#2326=ORIENTED_EDGE ( 'NONE', *, *, #4166, .F. ) ;
#2333=CARTESIAN_POINT ( 'NONE',  ( 2.708734125000000326, 112.3749999986344079, 1.121994411437819084 ) ) ;
#2335=ORIENTED_EDGE ( 'NONE', *, *, #1377, .T. ) ;
#2346=CARTESIAN_POINT ( 'NONE',  ( -1.915364268218909816, 110.9374999986344079, -1.915364268218909150 ) ) ;
#2351=EDGE_CURVE ( 'NONE', #7682, #7936, #6187, .T. ) ;
#2362=CARTESIAN_POINT ( 'NONE',  ( 3.980102097228898231E-16, 110.0000000000000000, -3.250000000000000444 ) ) ;
#2377=CARTESIAN_POINT ( 'NONE',  ( 2.708734124999999882, 110.6249999986343937, 1.121994411437818862 ) ) ;
#2387=DIRECTION ( 'NONE',  ( 0.000000000000000000, 0.000000000000000000, -1.000000000000000000 ) ) ;
#2392=CARTESIAN_POINT ( 'NONE',  ( -1.121994411437820194, 112.9999999986344079, -2.708734124999999882 ) ) ;
#2404=DIRECTION ( 'NONE',  ( 0.000000000000000000, 1.000000000000000000, 0.000000000000000000 ) ) ;
#2408=CARTESIAN_POINT ( 'NONE',  ( -4.975863863883684959E-16, 111.0624999986344079, -2.708734125000000326 ) ) ;
#2414=( BOUNDED_SURFACE ( )  B_SPLINE_SURFACE ( 1, 2, ( 
 ( #2874, #4810, #6804, #1943, #7851, #9713, #952, #6679, #1195, #4996, #1876, #2941, #3938, #6741, #2003, #8661, #4745, #11613, #3062, #2813, #3997, #6866, #11548, #10600, #1011, #9654, #7736, #1134, #5810, #2066, #4936, #5751, #8723, #6617, #8533, #3812, #10661, #2128, #7613, #9596, #2999, #1070, #11422, #9531, #184, #8783, #6925, #1253, #5061, #5991, #3122, #9779, #2180, #10720, #310, #8841, #4119, #11670, #3698, #4449, #10240, #11316, #12310, #12252, #9237 ),
 ( #2582, #5523, #1832, #10365, #10301, #3641, #10110, #723, #5642, #7507, #6569, #1652, #11190, #6515, #9419, #2762, #902, #5458, #4693, #655, #1770, #3581, #9298, #6449, #1590, #8486, #2526, #6389, #11065, #5393, #9174, #7448, #12130, #11254, #7389, #3760, #8247, #2642, #8308, #5581, #1715, #6326, #12068, #3524, #843, #7327, #785, #11126, #4572, #4516, #8366, #10177, #12193, #2703, #9359, #4635, #8428, #5765, #263, #1953, #9609, #2079, #136, #9545, #3076 ) ),
 .UNSPECIFIED., .F., .F., .F. ) 
 B_SPLINE_SURFACE_WITH_KNOTS ( ( 2, 2 ),
 ( 3, 2, 2, 2, 2, 2, 2, 2, 2, 2, 2, 2, 2, 2, 2, 2, 2, 2, 2, 2, 2, 2, 2, 2, 2, 2, 2, 2, 2, 2, 2, 2, 3 ),
 ( 0.000000000000000000, 1.000000000000000000 ),
 ( 0.000000000000000000, 0.03125000000000000000, 0.06250000000000000000, 0.09375000000000000000, 0.1250000000000000000, 0.1562500000000000000, 0.1875000000000000000, 0.2187500000000000000, 0.2500000000000000000, 0.2812500000000000000, 0.3125000000000000000, 0.3437500000000000000, 0.3750000000000000000, 0.4062500000000000000, 0.4375000000000000000, 0.4687500000000000000, 0.5000000000000000000, 0.5312500000000000000, 0.5625000000000000000, 0.5937500000000000000, 0.6250000000000000000, 0.6562500000000000000, 0.6875000000000000000, 0.7187500000000000000, 0.7500000000000000000, 0.7812500000000000000, 0.8125000000000000000, 0.8437500000000000000, 0.8750000000000000000, 0.9062500000000000000, 0.9375000000000000000, 0.9687500000000000000, 1.000000000000000000 ),
 .UNSPECIFIED. ) 
 GEOMETRIC_REPRESENTATION_ITEM ( )  RATIONAL_B_SPLINE_SURFACE ( (
 ( 1.000000000000000000, 0.9238795325112867385, 1.000000000000000000, 0.9238795325112867385, 1.000000000000000000, 0.9238795325112867385, 1.000000000000000000, 0.9238795325112867385, 1.000000000000000000, 0.9238795325112867385, 1.000000000000000000, 0.9238795325112867385, 1.000000000000000000, 0.9238795325112867385, 1.000000000000000000, 0.9238795325112867385, 1.000000000000000000, 0.9238795325112867385, 1.000000000000000000, 0.9238795325112867385, 1.000000000000000000, 0.9238795325112867385, 1.000000000000000000, 0.9238795325112867385, 1.000000000000000000, 0.9238795325112867385, 1.000000000000000000, 0.9238795325112867385, 1.000000000000000000, 0.9238795325112867385, 1.000000000000000000, 0.9238795325112867385, 1.000000000000000000, 0.9238795325112867385, 1.000000000000000000, 0.9238795325112867385, 1.000000000000000000, 0.9238795325112867385, 1.000000000000000000, 0.9238795325112867385, 1.000000000000000000, 0.9238795325112867385, 1.000000000000000000, 0.9238795325112867385, 1.000000000000000000, 0.9238795325112867385, 1.000000000000000000, 0.9238795325112867385, 1.000000000000000000, 0.9238795325112867385, 1.000000000000000000, 0.9238795325112867385, 1.000000000000000000, 0.9238795325112867385, 1.000000000000000000, 0.9238795325112867385, 1.000000000000000000, 0.9238795325112867385, 1.000000000000000000, 0.9238795325112867385, 1.000000000000000000, 0.9238795325112867385, 1.000000000000000000, 0.9238795325112867385, 1.000000000000000000),
 ( 1.000000000000000000, 0.9238795325112867385, 1.000000000000000000, 0.9238795325112867385, 1.000000000000000000, 0.9238795325112867385, 1.000000000000000000, 0.9238795325112867385, 1.000000000000000000, 0.9238795325112867385, 1.000000000000000000, 0.9238795325112867385, 1.000000000000000000, 0.9238795325112867385, 1.000000000000000000, 0.9238795325112867385, 1.000000000000000000, 0.9238795325112867385, 1.000000000000000000, 0.9238795325112867385, 1.000000000000000000, 0.9238795325112867385, 1.000000000000000000, 0.9238795325112867385, 1.000000000000000000, 0.9238795325112867385, 1.000000000000000000, 0.9238795325112867385, 1.000000000000000000, 0.9238795325112867385, 1.000000000000000000, 0.9238795325112867385, 1.000000000000000000, 0.9238795325112867385, 1.000000000000000000, 0.9238795325112867385, 1.000000000000000000, 0.9238795325112867385, 1.000000000000000000, 0.9238795325112867385, 1.000000000000000000, 0.9238795325112867385, 1.000000000000000000, 0.9238795325112867385, 1.000000000000000000, 0.9238795325112867385, 1.000000000000000000, 0.9238795325112867385, 1.000000000000000000, 0.9238795325112867385, 1.000000000000000000, 0.9238795325112867385, 1.000000000000000000, 0.9238795325112867385, 1.000000000000000000, 0.9238795325112867385, 1.000000000000000000, 0.9238795325112867385, 1.000000000000000000, 0.9238795325112867385, 1.000000000000000000, 0.9238795325112867385, 1.000000000000000000, 0.9238795325112867385, 1.000000000000000000) ) ) 
 REPRESENTATION_ITEM ( '' )  SURFACE ( )  );
#2418=VERTEX_POINT ( 'NONE', #1641 ) ;
#2424=VECTOR ( 'NONE', #3740, 1000.000000000000000 ) ;
#2430=EDGE_CURVE ( 'NONE', #9973, #9835, #3998, .T. ) ;
#2434=CARTESIAN_POINT ( 'NONE',  ( -2.298097038856279362, 114.2499999972688158, 2.298097038856279806 ) ) ;
#2447=CARTESIAN_POINT ( 'NONE',  ( -1.121994411437818862, 110.8749999986343937, 2.708734124999999882 ) ) ;
#2457=ORIENTED_EDGE ( 'NONE', *, *, #11720, .T. ) ;
#2460=CARTESIAN_POINT ( 'NONE',  ( -4.975863863883684959E-16, 112.0624999986344079, -2.708734125000000326 ) ) ;
#2470=EDGE_CURVE ( 'NONE', #7137, #7682, #5448, .T. ) ;
#2478=CARTESIAN_POINT ( 'NONE',  ( 1.658621287961228566E-16, 113.5624999986344079, 2.708734125000000326 ) ) ;
#2479=CARTESIAN_POINT ( 'NONE',  ( -2.708734124999999882, 111.0624999986344079, 3.317242575922456639E-16 ) ) ;
#2525=CARTESIAN_POINT ( 'NONE',  ( -1.121994411437820194, 111.9999999986343937, -2.708734124999999882 ) ) ;
#2526=CARTESIAN_POINT ( 'NONE',  ( -1.915364268218909594, 112.1874999986344079, -1.915364268218908927 ) ) ;
#2539=CARTESIAN_POINT ( 'NONE',  ( 1.346194077712559833, 111.8125000000000000, -3.250000000000000000 ) ) ;
#2546=CARTESIAN_POINT ( 'NONE',  ( 1.346194077712537629, 114.0624999972688016, 3.250000000000022649 ) ) ;
#2548=APPLICATION_CONTEXT ( 'automotive_design' ) ;
#2552=VERTEX_POINT ( 'NONE', #12184 ) ;
#2561=PRODUCT_DEFINITION_FORMATION_WITH_SPECIFIED_SOURCE ( 'ANY', '', #8763, .NOT_KNOWN. ) ;
#2576=VERTEX_POINT ( 'NONE', #10540 ) ;
#2579=CARTESIAN_POINT ( 'NONE',  ( 2.708734125000000326, 114.3124999986344079, 0.000000000000000000 ) ) ;
#2582=CARTESIAN_POINT ( 'NONE',  ( 2.708734124999999882, 110.5624999986344079, 0.000000000000000000 ) ) ;
#2598=CARTESIAN_POINT ( 'NONE',  ( 1.346194077712559389, 111.1875000000000142, 3.250000000000000444 ) ) ;
#2600=CARTESIAN_POINT ( 'NONE',  ( 2.708734125000000326, 110.3124999986344079, 0.000000000000000000 ) ) ;
#2629=CARTESIAN_POINT ( 'NONE',  ( 1.915364268218908705, 111.4374999986344079, -1.915364268218909594 ) ) ;
#2630=CARTESIAN_POINT ( 'NONE',  ( -5.970153145843347347E-16, 113.7500000000000000, -3.250000000000000444 ) ) ;
#2636=CARTESIAN_POINT ( 'NONE',  ( -3.250000000000000444, 112.4375000000000000, 1.346194077712559167 ) ) ;
#2638=ORIENTED_EDGE ( 'NONE', *, *, #4576, .F. ) ;
#2642=CARTESIAN_POINT ( 'NONE',  ( -1.121994411437818862, 112.8749999986344079, 2.708734124999999882 ) ) ;
#2654=CARTESIAN_POINT ( 'NONE',  ( -3.250000000000001776, 112.5625000000000000, -1.346194077712558723 ) ) ;
#2687=CARTESIAN_POINT ( 'NONE',  ( 2.708734124999999882, 113.6249999986344079, 1.121994411437818862 ) ) ;
#2691=EDGE_CURVE ( 'NONE', #9973, #8106, #10416, .T. ) ;
#2697=CARTESIAN_POINT ( 'NONE',  ( -3.250000000000000444, 112.5000000000000000, 3.980102097228898231E-16 ) ) ;
#2703=CARTESIAN_POINT ( 'NONE',  ( -1.121994411437818862, 113.8749999986343937, 2.708734124999999882 ) ) ;
#2704=CARTESIAN_POINT ( 'NONE',  ( 2.708734124999999882, 111.5624999986344079, 0.000000000000000000 ) ) ;
#2715=LINE ( 'NONE', #3886, #9451 ) ;
#2720=AXIS2_PLACEMENT_3D ( 'NONE', #2271, #8057, #2211 ) ;
#2726=CARTESIAN_POINT ( 'NONE',  ( -8.000000000000000000, 165.0000000000000000, -5.999999999999998224 ) ) ;
#2738=VERTEX_POINT ( 'NONE', #7047 ) ;
#2748=CARTESIAN_POINT ( 'NONE',  ( -1.121994411437820194, 111.2499999986344079, -2.708734124999999437 ) ) ;
#2754=VERTEX_POINT ( 'NONE', #7170 ) ;
#2762=CARTESIAN_POINT ( 'NONE',  ( 2.708734124999999437, 111.4999999986343937, -1.121994411437820638 ) ) ;
#2784=CARTESIAN_POINT ( 'NONE',  ( 3.249999999999999556, 112.9375000000000000, -1.346194077712561166 ) ) ;
#2792=CARTESIAN_POINT ( 'NONE',  ( -8.000000000000000000, 165.0000000000000000, 5.999999999999998224 ) ) ;
#2812=CARTESIAN_POINT ( 'NONE',  ( -2.708734125000000326, 114.1249999986344079, -1.121994411437818195 ) ) ;
#2813=CARTESIAN_POINT ( 'NONE',  ( 1.346194077712559389, 112.0624999972688016, 3.250000000000000444 ) ) ;
#2822=CARTESIAN_POINT ( 'NONE',  ( 0.000000000000000000, 110.0000000000000000, 0.000000000000000000 ) ) ;
#2854=DIRECTION ( 'NONE',  ( -0.000000000000000000, 1.000000000000000000, -0.000000000000000000 ) ) ;
#2872=CARTESIAN_POINT ( 'NONE',  ( 2.708734124999999882, 112.6249999986343937, 1.121994411437818862 ) ) ;
#2874=CARTESIAN_POINT ( 'NONE',  ( 3.250000000000000444, 110.8749999972688158, 0.000000000000000000 ) ) ;
#2887=CARTESIAN_POINT ( 'NONE',  ( 1.990051048614449116E-16, 113.2500000000000000, 3.250000000000000444 ) ) ;
#2889=CARTESIAN_POINT ( 'NONE',  ( -2.708734125000000326, 114.1249999986344079, -1.121994411437818195 ) ) ;
#2890=VECTOR ( 'NONE', #7348, 1000.000000000000000 ) ;
#2913=( BOUNDED_CURVE ( )  B_SPLINE_CURVE ( 2, ( #8119, #6202, #9994, #4448, #8246 ),
 .UNSPECIFIED., .F., .F. ) 
 B_SPLINE_CURVE_WITH_KNOTS ( ( 3, 2, 3 ),
 ( 0.9375000000000007772, 0.9687500000000004441, 1.000000000000000000 ),
 .UNSPECIFIED. ) 
 CURVE ( )  GEOMETRIC_REPRESENTATION_ITEM ( )  RATIONAL_B_SPLINE_CURVE ( ( 0.9999999999999981126, 0.9238795325112886259, 1.000000000000000000, 0.9238795325112867385, 1.000000000000000000 ) ) 
 REPRESENTATION_ITEM ( '' )  );
#2922=CARTESIAN_POINT ( 'NONE',  ( 0.000000000000000000, 115.0000000000000000, 0.000000000000000000 ) ) ;
#2930=VECTOR ( 'NONE', #10980, 1000.000000000000000 ) ;
#2933=CARTESIAN_POINT ( 'NONE',  ( 0.000000000000000000, 165.0000000000000000, 2.099999999999988987 ) ) ;
#2940=CARTESIAN_POINT ( 'NONE',  ( 1.121994411437819528, 114.1249999986344079, -2.708734124999999882 ) ) ;
#2941=CARTESIAN_POINT ( 'NONE',  ( -1.346194077712560944, 111.5624999972688300, -3.249999999999999556 ) ) ;
#2954=CARTESIAN_POINT ( 'NONE',  ( 1.346194077712559833, 110.8124999999999858, -3.250000000000000000 ) ) ;
#2956=CARTESIAN_POINT ( 'NONE',  ( -2.708734124999999882, 111.9999999986343937, 1.121994411437819084 ) ) ;
#2981=CARTESIAN_POINT ( 'NONE',  ( 0.000000000000000000, 165.0000000000000000, 0.000000000000000000 ) ) ;
#2983=VECTOR ( 'NONE', #5875, 1000.000000000000000 ) ;
#2987=DIRECTION ( 'NONE',  ( 0.8660254037844408170, -0.4999999999999961697, 0.000000000000000000 ) ) ;
#2998=CARTESIAN_POINT ( 'NONE',  ( -4.975863863883684959E-16, 112.0624999986344079, -2.708734125000000326 ) ) ;
#2999=CARTESIAN_POINT ( 'NONE',  ( -3.250000000000000444, 113.3749999972688158, 3.980102097228898231E-16 ) ) ;
#3010=CIRCLE ( 'NONE', #7779, 3.250000000000000444 ) ;
#3017=CIRCLE ( 'NONE', #9773, 2.099999999999988987 ) ;
#3018=CARTESIAN_POINT ( 'NONE',  ( -1.915364268218909594, 112.1874999986344079, -1.915364268218908927 ) ) ;
#3037=CARTESIAN_POINT ( 'NONE',  ( 2.298097038856279806, 113.1250000000000000, 2.298097038856279806 ) ) ;
#3041=DIRECTION ( 'NONE',  ( 0.000000000000000000, -1.000000000000000000, 0.000000000000000000 ) ) ;
#3049=LINE ( 'NONE', #10467, #6934 ) ;
#3052=CARTESIAN_POINT ( 'NONE',  ( 0.000000000000000000, 110.0000000000000000, 0.000000000000000000 ) ) ;
#3055=SHAPE_DEFINITION_REPRESENTATION ( #6681, #7136 ) ;
#3057=EDGE_CURVE ( 'NONE', #12307, #9534, #3049, .T. ) ;
#3062=CARTESIAN_POINT ( 'NONE',  ( 2.298097038856279806, 111.9999999972688158, 2.298097038856279806 ) ) ;
#3076=CARTESIAN_POINT ( 'NONE',  ( 2.708734124999999882, 114.5624999986344079, 0.000000000000000000 ) ) ;
#3078=CARTESIAN_POINT ( 'NONE',  ( -1.915364268218908927, 113.9374999986344079, 1.915364268218909150 ) ) ;
#3079=CONICAL_SURFACE ( 'NONE', #685, 2.099999999999998312, 1.029744258676656532 ) ;
#3081=ORIENTED_EDGE ( 'NONE', *, *, #2310, .F. ) ;
#3107=EDGE_CURVE ( 'NONE', #2738, #8492, #3798, .T. ) ;
#3108=CIRCLE ( 'NONE', #725, 9.999999999999998224 ) ;
#3114=CARTESIAN_POINT ( 'NONE',  ( -5.970153145843347347E-16, 111.6249999972688158, -3.250000000000000444 ) ) ;
#3121=CARTESIAN_POINT ( 'NONE',  ( -1.121994411437820416, 111.9999999986343937, -2.708734124999999882 ) ) ;
#3122=CARTESIAN_POINT ( 'NONE',  ( 2.298097038856279806, 113.9999999972688158, 2.298097038856279806 ) ) ;
#3138=CARTESIAN_POINT ( 'NONE',  ( -1.121994411437820194, 114.2499999986344079, -2.708734124999999437 ) ) ;
#3146=CARTESIAN_POINT ( 'NONE',  ( 0.000000000000000000, 165.0000000000000000, 0.000000000000000000 ) ) ;
#3161=CARTESIAN_POINT ( 'NONE',  ( 1.658621287961228566E-16, 112.5624999986344079, 2.708734125000000326 ) ) ;
#3169=EDGE_CURVE ( 'NONE', #9835, #8030, #1056, .T. ) ;
#3179=CARTESIAN_POINT ( 'NONE',  ( 2.708734125000000326, 113.3749999986344079, 1.121994411437818862 ) ) ;
#3188=EDGE_LOOP ( 'NONE', ( #2326, #2231, #8721, #9253, #1704, #11944 ) ) ;
#3212=CARTESIAN_POINT ( 'NONE',  ( -1.121994411437819084, 110.6249999986343937, 2.708734125000000326 ) ) ;
#3215=PRESENTATION_STYLE_ASSIGNMENT (( #2217 ) ) ;
#3219=FILL_AREA_STYLE_COLOUR ( '', #11286 ) ;
#3228=CARTESIAN_POINT ( 'NONE',  ( -1.121994411437818862, 113.6249999986344079, 2.708734125000000326 ) ) ;
#3233=EDGE_LOOP ( 'NONE', ( #12284, #8659, #6992, #1185 ) ) ;
#3256=VERTEX_POINT ( 'NONE', #6270 ) ;
#3267=CARTESIAN_POINT ( 'NONE',  ( -1.915364268218909150, 113.6874999986344079, 1.915364268218909594 ) ) ;
#3278=AXIS2_PLACEMENT_3D ( 'NONE', #3052, #6856, #7099 ) ;
#3282=CARTESIAN_POINT ( 'NONE',  ( 0.000000000000000000, 115.0000000000000000, 0.000000000000000000 ) ) ;
#3287=CARTESIAN_POINT ( 'NONE',  ( -1.915364268218909816, 112.9374999986344079, -1.915364268218909150 ) ) ;
#3297=CARTESIAN_POINT ( 'NONE',  ( -5.970153145843347347E-16, 113.6249999972688158, -3.250000000000000444 ) ) ;
#3303=CARTESIAN_POINT ( 'NONE',  ( -2.298097038856279806, 113.6250000000000000, -2.298097038856279362 ) ) ;
#3336=CARTESIAN_POINT ( 'NONE',  ( -4.975863863883684959E-16, 113.0624999986344079, -2.708734125000000326 ) ) ;
#3353=CARTESIAN_POINT ( 'NONE',  ( -2.708734125000000326, 113.7499999986343937, 1.121994411437818862 ) ) ;
#3359=( GEOMETRIC_REPRESENTATION_CONTEXT ( 3 ) GLOBAL_UNCERTAINTY_ASSIGNED_CONTEXT ( ( #4390 ) ) GLOBAL_UNIT_ASSIGNED_CONTEXT ( ( #1532, #6144, #8000 ) ) REPRESENTATION_CONTEXT ( 'NONE', 'WORKASPACE' ) );
#3372=DIRECTION ( 'NONE',  ( -0.000000000000000000, 1.000000000000000000, -0.000000000000000000 ) ) ;
#3382=CARTESIAN_POINT ( 'NONE',  ( 1.915364268218909150, 110.6874999986344079, 1.915364268218909150 ) ) ;
#3383=ADVANCED_FACE ( 'NONE', ( #11383 ), #1722, .T. ) ;
#3403=AXIS2_PLACEMENT_3D ( 'NONE', #1357, #7095, #7216 ) ;
#3416=CARTESIAN_POINT ( 'NONE',  ( 2.708734125000000326, 112.3124999986344079, 0.000000000000000000 ) ) ;
#3439=FACE_OUTER_BOUND ( 'NONE', #5328, .T. ) ;
#3446=DIRECTION ( 'NONE',  ( 0.000000000000000000, 0.000000000000000000, 1.000000000000000000 ) ) ;
#3450=VERTEX_POINT ( 'NONE', #1277 ) ;
#3460=CARTESIAN_POINT ( 'NONE',  ( 1.121994411437819528, 113.1249999986344079, -2.708734124999999882 ) ) ;
#3463=ORIENTED_EDGE ( 'NONE', *, *, #11291, .F. ) ;
#3469=FACE_OUTER_BOUND ( 'NONE', #9577, .T. ) ;
#3470=CARTESIAN_POINT ( 'NONE',  ( -8.000000000000000000, 115.0000000000000000, -5.999999999999998224 ) ) ;
#3475=CARTESIAN_POINT ( 'NONE',  ( 3.250000000000000444, 113.0625000000000000, 1.346194077712559389 ) ) ;
#3496=VECTOR ( 'NONE', #8006, 1000.000000000000000 ) ;
#3518=CARTESIAN_POINT ( 'NONE',  ( 1.346194077712564940, 110.8124999999999858, -3.249999999999993783 ) ) ;
#3523=CARTESIAN_POINT ( 'NONE',  ( 2.708734125000000326, 113.3124999986344079, 0.000000000000000000 ) ) ;
#3524=CARTESIAN_POINT ( 'NONE',  ( -1.121994411437820194, 113.2499999986344079, -2.708734124999999437 ) ) ;
#3538=CARTESIAN_POINT ( 'NONE',  ( -3.250000000000000444, 113.4375000000000000, 1.346194077712559389 ) ) ;
#3566=CARTESIAN_POINT ( 'NONE',  ( 2.708734125000000326, 110.3124999986344079, 0.000000000000000000 ) ) ;
#3567=DIRECTION ( 'NONE',  ( 0.000000000000000000, -0.000000000000000000, -1.000000000000000000 ) ) ;
#3581=CARTESIAN_POINT ( 'NONE',  ( -1.121994411437818862, 111.8749999986343937, 2.708734124999999882 ) ) ;
#3592=LINE ( 'NONE', #1417, #11388 ) ;
#3593=CARTESIAN_POINT ( 'NONE',  ( 3.250000000000000444, 111.0625000000000000, 1.346194077712559389 ) ) ;
#3627=CARTESIAN_POINT ( 'NONE',  ( -2.708734124999999882, 112.0624999986344079, 3.317242575922456639E-16 ) ) ;
#3641=CARTESIAN_POINT ( 'NONE',  ( -1.121994411437818862, 110.8749999986343937, 2.708734124999999882 ) ) ;
#3642=CARTESIAN_POINT ( 'NONE',  ( -1.915364268218908927, 110.9374999986344079, 1.915364268218909150 ) ) ;
#3685=CARTESIAN_POINT ( 'NONE',  ( -2.708734124999999882, 111.0624999986344079, 3.317242575922456639E-16 ) ) ;
#3698=CARTESIAN_POINT ( 'NONE',  ( -2.298097038856279806, 114.4999999972688158, -2.298097038856279362 ) ) ;
#3699=CARTESIAN_POINT ( 'NONE',  ( -2.708734124999999882, 110.9999999986343937, 1.121994411437819084 ) ) ;
#3714=ORIENTED_EDGE ( 'NONE', *, *, #348, .T. ) ;
#3723=CARTESIAN_POINT ( 'NONE',  ( 0.000000000000000000, 110.0000000000000000, 3.250000000000000444 ) ) ;
#3726=DIRECTION ( 'NONE',  ( -0.000000000000000000, 1.000000000000000000, -0.000000000000000000 ) ) ;
#3740=DIRECTION ( 'NONE',  ( -0.000000000000000000, -1.000000000000000000, -0.000000000000000000 ) ) ;
#3745=CARTESIAN_POINT ( 'NONE',  ( 1.121994411437818862, 113.7499999986343937, 2.708734124999999882 ) ) ;
#3753=CARTESIAN_POINT ( 'NONE',  ( -2.298097038856279362, 112.3750000000000000, 2.298097038856279806 ) ) ;
#3760=CARTESIAN_POINT ( 'NONE',  ( 1.121994411437818862, 112.7499999986343937, 2.708734124999999882 ) ) ;
#3779=AXIS2_PLACEMENT_3D ( 'NONE', #2141, #6631, #1025 ) ;
#3784=( BOUNDED_CURVE ( )  B_SPLINE_CURVE ( 2, ( #10690, #7822, #8872, #340, #11760, #3212, #1099, #2093, #4206, #6765, #2034, #5839, #8691, #3964, #5900, #9683, #1160, #4963, #10998, #6263, #8058, #4384, #11884, #11825, #11063, #7074, #1528, #2525, #2460, #10175, #7996, #525, #11125, #2333, #1587, #11941, #10053, #6325, #1466, #5331, #12066, #9108, #4322, #2392, #3336, #3460, #586, #7134, #3523, #9236, #8182, #5272, #12005, #7262, #3267, #10875, #10109, #5392, #5211, #10931, #9172, #653, #7326, #6141, #2579 ),
 .UNSPECIFIED., .F., .F. ) 
 B_SPLINE_CURVE_WITH_KNOTS ( ( 3, 2, 2, 2, 2, 2, 2, 2, 2, 2, 2, 2, 2, 2, 2, 2, 2, 2, 2, 2, 2, 2, 2, 2, 2, 2, 2, 2, 2, 2, 2, 2, 3 ),
 ( 0.000000000000000000, 0.03125000000000000000, 0.06250000000000000000, 0.09375000000000000000, 0.1250000000000000000, 0.1562500000000000000, 0.1875000000000000000, 0.2187500000000000000, 0.2500000000000000000, 0.2812500000000000000, 0.3125000000000000000, 0.3437500000000000000, 0.3750000000000000000, 0.4062500000000000000, 0.4375000000000000000, 0.4687500000000000000, 0.5000000000000000000, 0.5312500000000000000, 0.5625000000000000000, 0.5937500000000000000, 0.6250000000000000000, 0.6562500000000000000, 0.6875000000000000000, 0.7187500000000000000, 0.7500000000000000000, 0.7812500000000000000, 0.8125000000000000000, 0.8437500000000000000, 0.8750000000000000000, 0.9062500000000000000, 0.9375000000000000000, 0.9687500000000000000, 1.000000000000000000 ),
 .UNSPECIFIED. ) 
 CURVE ( )  GEOMETRIC_REPRESENTATION_ITEM ( )  RATIONAL_B_SPLINE_CURVE ( ( 1.000000000000000000, 0.9238795325112867385, 1.000000000000000000, 0.9238795325112867385, 1.000000000000000000, 0.9238795325112867385, 1.000000000000000000, 0.9238795325112867385, 1.000000000000000000, 0.9238795325112867385, 1.000000000000000000, 0.9238795325112867385, 1.000000000000000000, 0.9238795325112867385, 1.000000000000000000, 0.9238795325112867385, 1.000000000000000000, 0.9238795325112867385, 1.000000000000000000, 0.9238795325112867385, 1.000000000000000000, 0.9238795325112867385, 1.000000000000000000, 0.9238795325112867385, 1.000000000000000000, 0.9238795325112867385, 1.000000000000000000, 0.9238795325112867385, 1.000000000000000000, 0.9238795325112867385, 1.000000000000000000, 0.9238795325112867385, 1.000000000000000000, 0.9238795325112867385, 1.000000000000000000, 0.9238795325112867385, 1.000000000000000000, 0.9238795325112867385, 1.000000000000000000, 0.9238795325112867385, 1.000000000000000000, 0.9238795325112867385, 1.000000000000000000, 0.9238795325112867385, 1.000000000000000000, 0.9238795325112867385, 1.000000000000000000, 0.9238795325112867385, 1.000000000000000000, 0.9238795325112867385, 1.000000000000000000, 0.9238795325112867385, 1.000000000000000000, 0.9238795325112867385, 1.000000000000000000, 0.9238795325112867385, 1.000000000000000000, 0.9238795325112867385, 1.000000000000000000, 0.9238795325112867385, 1.000000000000000000, 0.9238795325112867385, 1.000000000000000000, 0.9238795325112867385, 1.000000000000000000 ) ) 
 REPRESENTATION_ITEM ( '' )  );
#3785=CARTESIAN_POINT ( 'NONE',  ( 0.000000000000000000, 165.0000000000000000, 0.000000000000000000 ) ) ;
#3792=ADVANCED_FACE ( 'NONE', ( #10728 ), #6748, .F. ) ;
#3798=LINE ( 'NONE', #7599, #1561 ) ;
#3806=CARTESIAN_POINT ( 'NONE',  ( 0.000000000000000000, 115.0000000000000000, 0.000000000000000000 ) ) ;
#3810=ORIENTED_EDGE ( 'NONE', *, *, #6550, .F. ) ;
#3811=CARTESIAN_POINT ( 'NONE',  ( -1.915364268218908927, 112.9374999986344079, 1.915364268218909150 ) ) ;
#3812=CARTESIAN_POINT ( 'NONE',  ( 1.346194077712559389, 113.0624999972688016, 3.250000000000000444 ) ) ;
#3829=CARTESIAN_POINT ( 'NONE',  ( -1.121994411437820194, 112.2499999986343937, -2.708734124999999437 ) ) ;
#3853=CARTESIAN_POINT ( 'NONE',  ( 0.000000000000000000, 110.0000000000000000, 3.250000000000000444 ) ) ;
#3854=DIRECTION ( 'NONE',  ( 0.000000000000000000, 0.000000000000000000, 1.000000000000000000 ) ) ;
#3870=DIRECTION ( 'NONE',  ( 0.000000000000000000, -0.000000000000000000, 1.000000000000000000 ) ) ;
#3871=AXIS2_PLACEMENT_3D ( 'NONE', #2822, #9478, #9293 ) ;
#3873=CARTESIAN_POINT ( 'NONE',  ( 1.915364268218908927, 114.1874999986344079, -1.915364268218909816 ) ) ;
#3886=CARTESIAN_POINT ( 'NONE',  ( -8.000000000000000000, 165.0000000000000000, -5.999999999999998224 ) ) ;
#3891=CARTESIAN_POINT ( 'NONE',  ( 3.249999999999999556, 112.9375000000000000, -1.346194077712561610 ) ) ;
#3904=CARTESIAN_POINT ( 'NONE',  ( 0.000000000000000000, 110.0000000000000000, 3.250000000000000444 ) ) ;
#3907=ORIENTED_EDGE ( 'NONE', *, *, #11654, .F. ) ;
#3918=ORIENTED_EDGE ( 'NONE', *, *, #8323, .T. ) ;
#3937=CARTESIAN_POINT ( 'NONE',  ( 2.708734124999999882, 113.2499999986344079, -1.121994411437820638 ) ) ;
#3938=CARTESIAN_POINT ( 'NONE',  ( -5.970153145843347347E-16, 111.6249999972688158, -3.250000000000000444 ) ) ;
#3948=CARTESIAN_POINT ( 'NONE',  ( -3.250000000000000444, 110.5000000000000000, 3.980102097228898231E-16 ) ) ;
#3953=ADVANCED_FACE ( 'NONE', ( #4305 ), #10789, .T. ) ;
#3954=CARTESIAN_POINT ( 'NONE',  ( -1.915364268218908927, 112.9374999986344079, 1.915364268218909150 ) ) ;
#3964=CARTESIAN_POINT ( 'NONE',  ( 1.121994411437819528, 111.1249999986343937, -2.708734124999999882 ) ) ;
#3967=AXIS2_PLACEMENT_3D ( 'NONE', #10687, #5089, #2150 ) ;
#3972=ORIENTED_EDGE ( 'NONE', *, *, #2430, .F. ) ;
#3977=CARTESIAN_POINT ( 'NONE',  ( -1.121994411437818862, 110.6249999986343937, 2.708734125000000326 ) ) ;
#3978=VECTOR ( 'NONE', #6479, 1000.000000000000000 ) ;
#3980=CARTESIAN_POINT ( 'NONE',  ( -1.346194077712573822, 113.1874999972688016, 3.249999999999985789 ) ) ;
#3996=CARTESIAN_POINT ( 'NONE',  ( 1.121994411437818862, 112.4999999986344079, 2.708734125000000326 ) ) ;
#3997=CARTESIAN_POINT ( 'NONE',  ( 1.990051048614449116E-16, 112.1249999972688158, 3.250000000000000444 ) ) ;
#3998=CIRCLE ( 'NONE', #5596, 2.099999999999998312 ) ;
#4007=CARTESIAN_POINT ( 'NONE',  ( -1.346194077712555837, 110.6875000000000000, -3.250000000000004885 ) ) ;
#4013=CARTESIAN_POINT ( 'NONE',  ( 2.708734124999999437, 113.4999999986344079, -1.121994411437820416 ) ) ;
#4017=EDGE_LOOP ( 'NONE', ( #11299, #4724, #4108, #5693 ) ) ;
#4040=DIRECTION ( 'NONE',  ( -0.000000000000000000, 1.000000000000000000, -0.000000000000000000 ) ) ;
#4044=CARTESIAN_POINT ( 'NONE',  ( -2.298097038856279806, 113.4999999972688158, -2.298097038856279362 ) ) ;
#4058=CARTESIAN_POINT ( 'NONE',  ( 1.915364268218908927, 111.1874999986344079, -1.915364268218909816 ) ) ;
#4059=VECTOR ( 'NONE', #4091, 1000.000000000000000 ) ;
#4060=FACE_OUTER_BOUND ( 'NONE', #7414, .T. ) ;
#4067=CARTESIAN_POINT ( 'NONE',  ( 0.000000000000000000, 165.0000000000000000, 0.000000000000000000 ) ) ;
#4077=CARTESIAN_POINT ( 'NONE',  ( -1.121994411437820194, 113.2499999986344079, -2.708734124999999437 ) ) ;
#4091=DIRECTION ( 'NONE',  ( -0.000000000000000000, 1.000000000000000000, -0.000000000000000000 ) ) ;
#4099=CARTESIAN_POINT ( 'NONE',  ( 2.708734124999999882, 111.2499999986344079, -1.121994411437820638 ) ) ;
#4103=EDGE_CURVE ( 'NONE', #11144, #8201, #11367, .T. ) ;
#4106=ORIENTED_EDGE ( 'NONE', *, *, #10124, .F. ) ;
#4108=ORIENTED_EDGE ( 'NONE', *, *, #8493, .T. ) ;
#4118=CARTESIAN_POINT ( 'NONE',  ( -1.915364268218909816, 112.9374999986344079, -1.915364268218909150 ) ) ;
#4119=CARTESIAN_POINT ( 'NONE',  ( -3.250000000000000444, 114.3749999972688158, 3.980102097228898231E-16 ) ) ;
#4126=ORIENTED_EDGE ( 'NONE', *, *, #3169, .T. ) ;
#4156=CARTESIAN_POINT ( 'NONE',  ( -1.346194077712559389, 110.3125000000000142, 3.250000000000000444 ) ) ;
#4161=LINE ( 'NONE', #5114, #12221 ) ;
#4163=CARTESIAN_POINT ( 'NONE',  ( -5.970153145843347347E-16, 112.6249999972688158, -3.250000000000000444 ) ) ;
#4166=EDGE_CURVE ( 'NONE', #5753, #9534, #10242, .T. ) ;
#4180=ORIENTED_EDGE ( 'NONE', *, *, #4410, .F. ) ;
#4206=CARTESIAN_POINT ( 'NONE',  ( -2.708734125000000326, 110.8124999986344079, 3.317242575922457132E-16 ) ) ;
#4211=SURFACE_STYLE_FILL_AREA ( #7706 ) ;
#4221=CARTESIAN_POINT ( 'NONE',  ( 2.708734124999999882, 112.2499999986344079, -1.121994411437820638 ) ) ;
#4223=CARTESIAN_POINT ( 'NONE',  ( 0.000000000000000000, 110.0000000000000000, 0.000000000000000000 ) ) ;
#4224=EDGE_CURVE ( 'NONE', #8106, #8030, #8444, .T. ) ;
#4228=DIRECTION ( 'NONE',  ( -0.000000000000000000, 1.000000000000000000, -0.000000000000000000 ) ) ;
#4233=ORIENTED_EDGE ( 'NONE', *, *, #11292, .T. ) ;
#4259=CARTESIAN_POINT ( 'NONE',  ( 3.250000000000000444, 111.0624999999999858, 1.346194077712559167 ) ) ;
#4261=EDGE_LOOP ( 'NONE', ( #3907, #3081, #4794, #9086 ) ) ;
#4267=EDGE_CURVE ( 'NONE', #11144, #3256, #4289, .T. ) ;
#4283=CARTESIAN_POINT ( 'NONE',  ( -1.121994411437820416, 111.9999999986343937, -2.708734124999999882 ) ) ;
#4285=DIRECTION ( 'NONE',  ( 0.000000000000000000, 0.000000000000000000, 1.000000000000000000 ) ) ;
#4289=LINE ( 'NONE', #8894, #9638 ) ;
#4297=CARTESIAN_POINT ( 'NONE',  ( -3.250000000000000444, 113.5000000000000000, 3.980102097228898231E-16 ) ) ;
#4305=FACE_OUTER_BOUND ( 'NONE', #3188, .T. ) ;
#4316=VERTEX_POINT ( 'NONE', #4163 ) ;
#4317=CARTESIAN_POINT ( 'NONE',  ( 0.000000000000000000, 110.0000000000000000, 3.250000000000000444 ) ) ;
#4322=CARTESIAN_POINT ( 'NONE',  ( -1.915364268218909816, 112.9374999986344079, -1.915364268218909150 ) ) ;
#4326=ORIENTED_EDGE ( 'NONE', *, *, #11083, .F. ) ;
#4331=CARTESIAN_POINT ( 'NONE',  ( -8.000000000000000000, 165.0000000000000000, -5.999999999999998224 ) ) ;
#4338=CARTESIAN_POINT ( 'NONE',  ( 1.121994411437818862, 112.4999999986344079, 2.708734125000000326 ) ) ;
#4339=CARTESIAN_POINT ( 'NONE',  ( -2.708734125000000326, 111.1249999986343937, -1.121994411437818195 ) ) ;
#4350=CYLINDRICAL_SURFACE ( 'NONE', #12147, 3.250000000000000444 ) ;
#4366=CARTESIAN_POINT ( 'NONE',  ( 0.000000000000000000, 165.0000000000000000, 0.000000000000000000 ) ) ;
#4375=CARTESIAN_POINT ( 'NONE',  ( 1.346194077712550063, 112.0624999972687590, 3.250000000000008438 ) ) ;
#4377=ORIENTED_EDGE ( 'NONE', *, *, #10723, .T. ) ;
#4384=CARTESIAN_POINT ( 'NONE',  ( -1.121994411437819084, 111.6249999986343937, 2.708734125000000326 ) ) ;
#4390=UNCERTAINTY_MEASURE_WITH_UNIT (LENGTH_MEASURE( 1.000000000000000082E-05 ), #1532, 'distance_accuracy_value', 'NONE');
#4401=CARTESIAN_POINT ( 'NONE',  ( 3.250000000000000444, 114.0000000000000000, 0.000000000000000000 ) ) ;
#4410=EDGE_CURVE ( 'NONE', #1153, #6351, #804, .T. ) ;
#4412=CARTESIAN_POINT ( 'NONE',  ( 1.346194077712578041, 113.6874999972688300, -3.249999999999981792 ) ) ;
#4416=CARTESIAN_POINT ( 'NONE',  ( 0.000000000000000000, 110.0000000000000000, 0.000000000000000000 ) ) ;
#4436=DIRECTION ( 'NONE',  ( 0.000000000000000000, 0.000000000000000000, -1.000000000000000000 ) ) ;
#4437=ORIENTED_EDGE ( 'NONE', *, *, #196, .T. ) ;
#4438=DIRECTION ( 'NONE',  ( 0.000000000000000000, 0.000000000000000000, 1.000000000000000000 ) ) ;
#4448=CARTESIAN_POINT ( 'NONE',  ( 3.249999999999999556, 114.8124999972688016, -1.346194077712561166 ) ) ;
#4449=CARTESIAN_POINT ( 'NONE',  ( -1.346194077712560944, 114.5624999972688300, -3.249999999999999556 ) ) ;
#4466=CARTESIAN_POINT ( 'NONE',  ( 3.249999999999999556, 110.9374999999999858, -1.346194077712561610 ) ) ;
#4471=CONICAL_SURFACE ( 'NONE', #11455, 2.099999999999998312, 1.029744258676656532 ) ;
#4476=ORIENTED_EDGE ( 'NONE', *, *, #8878, .F. ) ;
#4490=( BOUNDED_CURVE ( )  B_SPLINE_CURVE ( 2, ( #7072, #5150, #8928, #398, #9928, #10625, #7933, #5025, #6828 ),
 .UNSPECIFIED., .F., .F. ) 
 B_SPLINE_CURVE_WITH_KNOTS ( ( 3, 2, 2, 2, 3 ),
 ( 0.3125000000000002776, 0.3437500000000003331, 0.3750000000000003331, 0.4062500000000003331, 0.4375000000000003886 ),
 .UNSPECIFIED. ) 
 CURVE ( )  GEOMETRIC_REPRESENTATION_ITEM ( )  RATIONAL_B_SPLINE_CURVE ( ( 0.9999999999999993339, 0.9238795325112874046, 1.000000000000000000, 0.9238795325112867385, 1.000000000000000000, 0.9238795325112867385, 1.000000000000000000, 0.9238795325112857393, 1.000000000000000888 ) ) 
 REPRESENTATION_ITEM ( '' )  );
#4500=CARTESIAN_POINT ( 'NONE',  ( 1.990051048614449116E-16, 111.1249999972688158, 3.250000000000000444 ) ) ;
#4516=CARTESIAN_POINT ( 'NONE',  ( 2.708734124999999882, 113.6249999986344079, 1.121994411437818862 ) ) ;
#4531=CARTESIAN_POINT ( 'NONE',  ( -5.970153145843347347E-16, 110.7500000000000000, -3.250000000000000444 ) ) ;
#4558=CARTESIAN_POINT ( 'NONE',  ( 1.915364268218909150, 111.6874999986344079, 1.915364268218909150 ) ) ;
#4566=ORIENTED_EDGE ( 'NONE', *, *, #4224, .T. ) ;
#4572=CARTESIAN_POINT ( 'NONE',  ( 2.708734124999999882, 113.5624999986344079, 0.000000000000000000 ) ) ;
#4573=CARTESIAN_POINT ( 'NONE',  ( 1.915364268218908705, 111.4374999986344079, -1.915364268218909594 ) ) ;
#4576=EDGE_CURVE ( 'NONE', #9884, #2552, #9175, .T. ) ;
#4577=EDGE_CURVE ( 'NONE', #7882, #2552, #12334, .T. ) ;
#4588=CARTESIAN_POINT ( 'NONE',  ( 3.250000000000000444, 111.0000000000000000, 0.000000000000000000 ) ) ;
#4608=AXIS2_PLACEMENT_3D ( 'NONE', #11645, #8816, #6092 ) ;
#4620=CARTESIAN_POINT ( 'NONE',  ( 2.708734124999999437, 113.4999999986344079, -1.121994411437820638 ) ) ;
#4625=EDGE_LOOP ( 'NONE', ( #9747, #529, #9005, #4999, #324, #2638, #6306, #9540, #7157, #7425, #2116, #8824 ) ) ;
#4635=CARTESIAN_POINT ( 'NONE',  ( -2.708734124999999882, 113.9999999986343937, 1.121994411437818862 ) ) ;
#4637=EDGE_CURVE ( 'NONE', #6351, #7137, #6480, .T. ) ;
#4678=CARTESIAN_POINT ( 'NONE',  ( 0.000000000000000000, 115.0000000000000000, 0.000000000000000000 ) ) ;
#4681=CARTESIAN_POINT ( 'NONE',  ( -2.708734124999999882, 113.0624999986344079, 3.317242575922456639E-16 ) ) ;
#4682=PLANE ( 'NONE',  #217 ) ;
#4693=CARTESIAN_POINT ( 'NONE',  ( 1.915364268218909150, 111.6874999986344079, 1.915364268218909150 ) ) ;
#4699=VERTEX_POINT ( 'NONE', #7088 ) ;
#4704=CARTESIAN_POINT ( 'NONE',  ( 1.224646799147353059E-15, 115.0000000000000000, 9.999999999999998224 ) ) ;
#4724=ORIENTED_EDGE ( 'NONE', *, *, #9813, .T. ) ;
#4726=EDGE_CURVE ( 'NONE', #2418, #12307, #9880, .T. ) ;
#4736=CARTESIAN_POINT ( 'NONE',  ( 3.250000000000000444, 114.4374999986344079, 0.000000000000000000 ) ) ;
#4741=CARTESIAN_POINT ( 'NONE',  ( 2.708734124999999437, 111.4999999986343937, -1.121994411437820638 ) ) ;
#4745=CARTESIAN_POINT ( 'NONE',  ( 3.250000000000000444, 111.8749999972688158, 0.000000000000000000 ) ) ;
#4759=CARTESIAN_POINT ( 'NONE',  ( -2.708734124999999882, 113.9999999986344079, 1.121994411437819084 ) ) ;
#4772=VECTOR ( 'NONE', #11405, 1000.000000000000114 ) ;
#4785=CARTESIAN_POINT ( 'NONE',  ( 0.000000000000000000, 115.0000000000000000, 3.250000000000000444 ) ) ;
#4786=CARTESIAN_POINT ( 'NONE',  ( 2.979367062500000163, 114.7187499979516190, 0.000000000000000000 ) ) ;
#4794=ORIENTED_EDGE ( 'NONE', *, *, #5822, .T. ) ;
#4807=EDGE_CURVE ( 'NONE', #5440, #11360, #663, .T. ) ;
#4809=CARTESIAN_POINT ( 'NONE',  ( -1.121994411437818862, 113.8749999986343937, 2.708734124999999882 ) ) ;
#4810=CARTESIAN_POINT ( 'NONE',  ( 3.250000000000000444, 110.9374999972688016, 1.346194077712559389 ) ) ;
#4826=CARTESIAN_POINT ( 'NONE',  ( 1.121994411437819084, 112.7499999986344079, 2.708734124999999882 ) ) ;
#4840=( NAMED_UNIT ( * ) PLANE_ANGLE_UNIT ( ) SI_UNIT ( $, .RADIAN. ) );
#4872=ORIENTED_EDGE ( 'NONE', *, *, #4577, .T. ) ;
#4873=CARTESIAN_POINT ( 'NONE',  ( -1.121994411437818862, 112.6249999986343937, 2.708734125000000326 ) ) ;
#4892=ORIENTED_EDGE ( 'NONE', *, *, #7315, .F. ) ;
#4907=EDGE_CURVE ( 'NONE', #1153, #5440, #2715, .T. ) ;
#4935=CARTESIAN_POINT ( 'NONE',  ( -4.975863863883684959E-16, 113.0624999986344079, -2.708734125000000326 ) ) ;
#4936=CARTESIAN_POINT ( 'NONE',  ( 2.298097038856278918, 112.7499999972688158, -2.298097038856279806 ) ) ;
#4947=CARTESIAN_POINT ( 'NONE',  ( -3.250000000000000444, 110.4375000000000000, 1.346194077712559167 ) ) ;
#4948=DIRECTION ( 'NONE',  ( 1.049727191138619928E-16, 0.5150380749100523792, -0.8571673007021134438 ) ) ;
#4951=DIRECTION ( 'NONE',  ( -1.000000000000000000, 0.000000000000000000, -0.000000000000000000 ) ) ;
#4952=CARTESIAN_POINT ( 'NONE',  ( 1.121994411437819084, 113.3749999986344079, -2.708734124999999437 ) ) ;
#4963=CARTESIAN_POINT ( 'NONE',  ( 2.708734125000000326, 111.3749999986344079, 1.121994411437819084 ) ) ;
#4967=ADVANCED_FACE ( 'NONE', ( #9789 ), #6936, .T. ) ;
#4989=EDGE_CURVE ( 'NONE', #3450, #5494, #6643, .T. ) ;
#4995=CARTESIAN_POINT ( 'NONE',  ( 1.121994411437819528, 113.1249999986343937, -2.708734124999999882 ) ) ;
#4996=CARTESIAN_POINT ( 'NONE',  ( -3.250000000000001776, 111.4374999972688300, -1.346194077712558723 ) ) ;
#4999=ORIENTED_EDGE ( 'NONE', *, *, #153, .F. ) ;
#5002=ORIENTED_EDGE ( 'NONE', *, *, #11083, .T. ) ;
#5016=CARTESIAN_POINT ( 'NONE',  ( 2.708734124999999882, 112.5624999986344079, 0.000000000000000000 ) ) ;
#5025=CARTESIAN_POINT ( 'NONE',  ( -1.346194077712548287, 112.5624999972688016, -3.250000000000012434 ) ) ;
#5032=DIRECTION ( 'NONE',  ( 1.000000000000000000, 0.000000000000000000, 0.000000000000000000 ) ) ;
#5042=CARTESIAN_POINT ( 'NONE',  ( 1.121994411437818862, 111.4999999986343937, 2.708734125000000326 ) ) ;
#5043=AXIS2_PLACEMENT_3D ( 'NONE', #11295, #1686, #12226 ) ;
#5045=CARTESIAN_POINT ( 'NONE',  ( -3.250000000000001776, 113.4374999972688300, -1.346194077712558279 ) ) ;
#5047=( BOUNDED_CURVE ( )  B_SPLINE_CURVE ( 2, ( #6260, #3518, #11120, #1395, #454, #4259, #9988, #7128, #1459 ),
 .UNSPECIFIED., .F., .F. ) 
 B_SPLINE_CURVE_WITH_KNOTS ( ( 3, 2, 2, 2, 3 ),
 ( 0.1875000000000001665, 0.2187500000000001943, 0.2500000000000002220, 0.2812500000000002220, 0.3125000000000002776 ),
 .UNSPECIFIED. ) 
 CURVE ( )  GEOMETRIC_REPRESENTATION_ITEM ( )  RATIONAL_B_SPLINE_CURVE ( ( 0.9999999999999995559, 0.9238795325112871826, 1.000000000000000000, 0.9238795325112867385, 1.000000000000000000, 0.9238795325112867385, 1.000000000000000000, 0.9238795325112860723, 1.000000000000000666 ) ) 
 REPRESENTATION_ITEM ( '' )  );
#5048=PRODUCT_DEFINITION ( 'UNKNOWN', '', #2561, #7007 ) ;
#5053=DIRECTION ( 'NONE',  ( -0.000000000000000000, 1.000000000000000000, -0.000000000000000000 ) ) ;
#5055=ORIENTED_EDGE ( 'NONE', *, *, #4637, .T. ) ;
#5057=PLANE ( 'NONE',  #16 ) ;
#5059=CARTESIAN_POINT ( 'NONE',  ( -1.915364268218909816, 110.9374999986344079, -1.915364268218909150 ) ) ;
#5061=CARTESIAN_POINT ( 'NONE',  ( 3.250000000000000444, 113.8749999972688158, 0.000000000000000000 ) ) ;
#5065=ORIENTED_EDGE ( 'NONE', *, *, #11848, .F. ) ;
#5074=( BOUNDED_SURFACE ( )  B_SPLINE_SURFACE ( 1, 2, ( 
 ( #6659, #232, #10700, #103, #167, #3977, #5732, #7654, #1115, #10947, #2346, #289, #2408, #7092, #11838, #4099, #9066, #10010, #7890, #5042, #7150, #11012, #1295, #1355, #9943, #5106, #8823, #4283, #11709, #10889, #8077, #4221, #3416, #1235, #6098, #4338, #3161, #6219, #5164, #8012, #11901, #7025, #3287, #5289, #2227, #8943, #6964, #1481, #9821, #6034, #6153, #10767, #2478, #3228, #1419, #3353, #416, #9883, #5227, #9003, #478, #540, #8886, #350, #7213 ),
 ( #8135, #11956, #11778, #6278, #10825, #4156, #7948, #2288, #11437, #8383, #10492, #10256, #4531, #2954, #8615, #4466, #4588, #3593, #7405, #2598, #12019, #10192, #11503, #8196, #74, #1730, #1604, #10069, #12087, #2539, #9254, #11139, #8262, #10127, #796, #7341, #5766, #7688, #1544, #5412, #5536, #2654, #13, #9189, #668, #1664, #9546, #3891, #738, #3475, #6341, #605, #2887, #6696, #5347, #3538, #6405, #1026, #9315, #8321, #12144, #5473, #1954, #11205, #4401 ) ),
 .UNSPECIFIED., .F., .F., .T. ) 
 B_SPLINE_SURFACE_WITH_KNOTS ( ( 2, 2 ),
 ( 3, 2, 2, 2, 2, 2, 2, 2, 2, 2, 2, 2, 2, 2, 2, 2, 2, 2, 2, 2, 2, 2, 2, 2, 2, 2, 2, 2, 2, 2, 2, 2, 3 ),
 ( 0.000000000000000000, 1.000000000000000000 ),
 ( 0.000000000000000000, 0.03125000000000000000, 0.06250000000000000000, 0.09375000000000000000, 0.1250000000000000000, 0.1562500000000000000, 0.1875000000000000000, 0.2187500000000000000, 0.2500000000000000000, 0.2812500000000000000, 0.3125000000000000000, 0.3437500000000000000, 0.3750000000000000000, 0.4062500000000000000, 0.4375000000000000000, 0.4687500000000000000, 0.5000000000000000000, 0.5312500000000000000, 0.5625000000000000000, 0.5937500000000000000, 0.6250000000000000000, 0.6562500000000000000, 0.6875000000000000000, 0.7187500000000000000, 0.7500000000000000000, 0.7812500000000000000, 0.8125000000000000000, 0.8437500000000000000, 0.8750000000000000000, 0.9062500000000000000, 0.9375000000000000000, 0.9687500000000000000, 1.000000000000000000 ),
 .UNSPECIFIED. ) 
 GEOMETRIC_REPRESENTATION_ITEM ( )  RATIONAL_B_SPLINE_SURFACE ( (
 ( 1.000000000000000000, 0.9238795325112867385, 1.000000000000000000, 0.9238795325112867385, 1.000000000000000000, 0.9238795325112867385, 1.000000000000000000, 0.9238795325112867385, 1.000000000000000000, 0.9238795325112867385, 1.000000000000000000, 0.9238795325112867385, 1.000000000000000000, 0.9238795325112867385, 1.000000000000000000, 0.9238795325112867385, 1.000000000000000000, 0.9238795325112867385, 1.000000000000000000, 0.9238795325112867385, 1.000000000000000000, 0.9238795325112867385, 1.000000000000000000, 0.9238795325112867385, 1.000000000000000000, 0.9238795325112867385, 1.000000000000000000, 0.9238795325112867385, 1.000000000000000000, 0.9238795325112867385, 1.000000000000000000, 0.9238795325112867385, 1.000000000000000000, 0.9238795325112867385, 1.000000000000000000, 0.9238795325112867385, 1.000000000000000000, 0.9238795325112867385, 1.000000000000000000, 0.9238795325112867385, 1.000000000000000000, 0.9238795325112867385, 1.000000000000000000, 0.9238795325112867385, 1.000000000000000000, 0.9238795325112867385, 1.000000000000000000, 0.9238795325112867385, 1.000000000000000000, 0.9238795325112867385, 1.000000000000000000, 0.9238795325112867385, 1.000000000000000000, 0.9238795325112867385, 1.000000000000000000, 0.9238795325112867385, 1.000000000000000000, 0.9238795325112867385, 1.000000000000000000, 0.9238795325112867385, 1.000000000000000000, 0.9238795325112867385, 1.000000000000000000, 0.9238795325112867385, 1.000000000000000000),
 ( 1.000000000000000000, 0.9238795325112867385, 1.000000000000000000, 0.9238795325112867385, 1.000000000000000000, 0.9238795325112867385, 1.000000000000000000, 0.9238795325112867385, 1.000000000000000000, 0.9238795325112867385, 1.000000000000000000, 0.9238795325112867385, 1.000000000000000000, 0.9238795325112867385, 1.000000000000000000, 0.9238795325112867385, 1.000000000000000000, 0.9238795325112867385, 1.000000000000000000, 0.9238795325112867385, 1.000000000000000000, 0.9238795325112867385, 1.000000000000000000, 0.9238795325112867385, 1.000000000000000000, 0.9238795325112867385, 1.000000000000000000, 0.9238795325112867385, 1.000000000000000000, 0.9238795325112867385, 1.000000000000000000, 0.9238795325112867385, 1.000000000000000000, 0.9238795325112867385, 1.000000000000000000, 0.9238795325112867385, 1.000000000000000000, 0.9238795325112867385, 1.000000000000000000, 0.9238795325112867385, 1.000000000000000000, 0.9238795325112867385, 1.000000000000000000, 0.9238795325112867385, 1.000000000000000000, 0.9238795325112867385, 1.000000000000000000, 0.9238795325112867385, 1.000000000000000000, 0.9238795325112867385, 1.000000000000000000, 0.9238795325112867385, 1.000000000000000000, 0.9238795325112867385, 1.000000000000000000, 0.9238795325112867385, 1.000000000000000000, 0.9238795325112867385, 1.000000000000000000, 0.9238795325112867385, 1.000000000000000000, 0.9238795325112867385, 1.000000000000000000, 0.9238795325112867385, 1.000000000000000000) ) ) 
 REPRESENTATION_ITEM ( '' )  SURFACE ( )  );
#5084=EDGE_LOOP ( 'NONE', ( #10237, #9646, #8203, #4106 ) ) ;
#5089=DIRECTION ( 'NONE',  ( 0.000000000000000000, 1.000000000000000000, 0.000000000000000000 ) ) ;
#5094=ORIENTED_EDGE ( 'NONE', *, *, #1377, .F. ) ;
#5097=AXIS2_PLACEMENT_3D ( 'NONE', #3785, #5846, #11524 ) ;
#5106=CARTESIAN_POINT ( 'NONE',  ( -2.708734125000000770, 111.8749999986343937, -1.121994411437818639 ) ) ;
#5114=CARTESIAN_POINT ( 'NONE',  ( 0.000000000000000000, 153.0000000000000000, 2.099999999999998312 ) ) ;
#5122=DIRECTION ( 'NONE',  ( -0.000000000000000000, 1.000000000000000000, -0.000000000000000000 ) ) ;
#5123=VERTEX_POINT ( 'NONE', #11989 ) ;
#5124=CARTESIAN_POINT ( 'NONE',  ( -1.346194077712581150, 113.3125000000000000, 3.249999999999978240 ) ) ;
#5150=CARTESIAN_POINT ( 'NONE',  ( -1.346194077712568049, 112.1874999972688016, 3.249999999999991118 ) ) ;
#5164=CARTESIAN_POINT ( 'NONE',  ( -1.915364268218909150, 112.6874999986344079, 1.915364268218909594 ) ) ;
#5167=FACE_BOUND ( 'NONE', #9826, .T. ) ;
#5180=CARTESIAN_POINT ( 'NONE',  ( -1.346194077712535409, 113.6875000000000000, -3.250000000000024869 ) ) ;
#5211=CARTESIAN_POINT ( 'NONE',  ( -1.915364268218909816, 113.9374999986344079, -1.915364268218909150 ) ) ;
#5214=EDGE_LOOP ( 'NONE', ( #8417, #4437, #1462, #9926 ) ) ;
#5224=DIRECTION ( 'NONE',  ( 0.000000000000000000, 0.000000000000000000, 1.000000000000000000 ) ) ;
#5227=CARTESIAN_POINT ( 'NONE',  ( -1.915364268218909816, 113.9374999986344079, -1.915364268218909150 ) ) ;
#5231=DIRECTION ( 'NONE',  ( 0.000000000000000000, 0.5150380749100523792, 0.8571673007021134438 ) ) ;
#5233=DIRECTION ( 'NONE',  ( 0.000000000000000000, 0.000000000000000000, 1.000000000000000000 ) ) ;
#5272=CARTESIAN_POINT ( 'NONE',  ( 1.121994411437819084, 113.4999999986344079, 2.708734125000000326 ) ) ;
#5289=CARTESIAN_POINT ( 'NONE',  ( -1.121994411437820416, 112.9999999986343937, -2.708734124999999882 ) ) ;
#5290=CARTESIAN_POINT ( 'NONE',  ( 1.915364268218909150, 110.6874999986344079, 1.915364268218909150 ) ) ;
#5302=ORIENTED_EDGE ( 'NONE', *, *, #348, .F. ) ;
#5306=DIRECTION ( 'NONE',  ( 0.000000000000000000, 0.000000000000000000, 1.000000000000000000 ) ) ;
#5308=ORIENTED_EDGE ( 'NONE', *, *, #2430, .T. ) ;
#5317=CARTESIAN_POINT ( 'NONE',  ( 1.346194077712544956, 112.1875000000000142, 3.250000000000015543 ) ) ;
#5328=EDGE_LOOP ( 'NONE', ( #6807, #5450, #9890, #5831 ) ) ;
#5331=CARTESIAN_POINT ( 'NONE',  ( -2.708734125000000326, 112.7499999986344079, 1.121994411437819084 ) ) ;
#5335=EDGE_LOOP ( 'NONE', ( #772, #7737, #3714 ) ) ;
#5343=CARTESIAN_POINT ( 'NONE',  ( 2.571758278209439492E-16, 153.0000000000000000, -2.099999999999998312 ) ) ;
#5347=CARTESIAN_POINT ( 'NONE',  ( -2.298097038856279362, 113.3750000000000000, 2.298097038856279806 ) ) ;
#5349=DIRECTION ( 'NONE',  ( -0.000000000000000000, 1.000000000000000000, -0.000000000000000000 ) ) ;
#5367=CARTESIAN_POINT ( 'NONE',  ( -1.346194077712535409, 114.5624999972688158, -3.250000000000024869 ) ) ;
#5377=CARTESIAN_POINT ( 'NONE',  ( 3.250000000000000444, 112.0624999999999858, 1.346194077712559167 ) ) ;
#5378=CARTESIAN_POINT ( 'NONE',  ( 0.000000000000000000, 110.0000000000000000, 0.000000000000000000 ) ) ;
#5382=EDGE_CURVE ( 'NONE', #5829, #5123, #8846, .T. ) ;
#5392=CARTESIAN_POINT ( 'NONE',  ( -2.708734125000000770, 113.8749999986344079, -1.121994411437818639 ) ) ;
#5393=CARTESIAN_POINT ( 'NONE',  ( 1.121994411437819084, 112.3749999986344221, -2.708734124999999437 ) ) ;
#5395=( BOUNDED_CURVE ( )  B_SPLINE_CURVE ( 2, ( #291, #3980, #1053, #995, #11595, #5045, #4044, #6847, #6784 ),
 .UNSPECIFIED., .F., .F. ) 
 B_SPLINE_CURVE_WITH_KNOTS ( ( 3, 2, 2, 2, 3 ),
 ( 0.5625000000000004441, 0.5937500000000004441, 0.6250000000000004441, 0.6562500000000005551, 0.6875000000000005551 ),
 .UNSPECIFIED. ) 
 CURVE ( )  GEOMETRIC_REPRESENTATION_ITEM ( )  RATIONAL_B_SPLINE_CURVE ( ( 0.9999999999999988898, 0.9238795325112878487, 1.000000000000000000, 0.9238795325112867385, 1.000000000000000000, 0.9238795325112867385, 1.000000000000000000, 0.9238795325112854062, 1.000000000000001332 ) ) 
 REPRESENTATION_ITEM ( '' )  );
#5410=CARTESIAN_POINT ( 'NONE',  ( 3.249999999999999556, 111.8124999972688016, -1.346194077712561166 ) ) ;
#5412=CARTESIAN_POINT ( 'NONE',  ( -3.250000000000000444, 112.4375000000000000, 1.346194077712559389 ) ) ;
#5438=CARTESIAN_POINT ( 'NONE',  ( 3.250000000000000444, 110.4374999986344079, 0.000000000000000000 ) ) ;
#5440=VERTEX_POINT ( 'NONE', #5987 ) ;
#5448=LINE ( 'NONE', #11245, #6957 ) ;
#5450=ORIENTED_EDGE ( 'NONE', *, *, #9367, .T. ) ;
#5458=CARTESIAN_POINT ( 'NONE',  ( 2.708734124999999882, 111.6249999986344079, 1.121994411437818862 ) ) ;
#5473=CARTESIAN_POINT ( 'NONE',  ( 1.346194077712559833, 113.8125000000000000, -3.250000000000000000 ) ) ;
#5486=AXIS2_PLACEMENT_3D ( 'NONE', #5885, #5820, #9605 ) ;
#5494=VERTEX_POINT ( 'NONE', #11851 ) ;
#5504=CARTESIAN_POINT ( 'NONE',  ( 2.298097038856279806, 110.9999999972688158, 2.298097038856279806 ) ) ;
#5508=CARTESIAN_POINT ( 'NONE',  ( -4.975863863883684959E-16, 111.3124999986344079, -2.708734124999999882 ) ) ;
#5517=CYLINDRICAL_SURFACE ( 'NONE', #3871, 3.250000000000000444 ) ;
#5523=CARTESIAN_POINT ( 'NONE',  ( 2.708734124999999882, 110.6249999986343937, 1.121994411437818862 ) ) ;
#5529=DIRECTION ( 'NONE',  ( -0.000000000000000000, 1.000000000000000000, -0.000000000000000000 ) ) ;
#5536=CARTESIAN_POINT ( 'NONE',  ( -3.250000000000000444, 112.5000000000000000, 3.980102097228898231E-16 ) ) ;
#5561=EDGE_CURVE ( 'NONE', #7137, #1550, #9825, .T. ) ;
#5566=CARTESIAN_POINT ( 'NONE',  ( 1.121994411437819084, 113.3749999986344079, -2.708734124999999437 ) ) ;
#5568=CARTESIAN_POINT ( 'NONE',  ( 3.980102097228898231E-16, 110.0000000000000000, -3.250000000000000444 ) ) ;
#5581=CARTESIAN_POINT ( 'NONE',  ( -2.708734124999999882, 112.9999999986343937, 1.121994411437818862 ) ) ;
#5596=AXIS2_PLACEMENT_3D ( 'NONE', #9410, #10353, #4438 ) ;
#5599=ADVANCED_FACE ( 'NONE', ( #7162 ), #3079, .F. ) ;
#5628=CARTESIAN_POINT ( 'NONE',  ( -1.915364268218909594, 113.1874999986344079, -1.915364268218908927 ) ) ;
#5642=CARTESIAN_POINT ( 'NONE',  ( -2.708734124999999882, 111.0624999986344079, 3.317242575922456639E-16 ) ) ;
#5666=CARTESIAN_POINT ( 'NONE',  ( -5.970153145843347347E-16, 112.7500000000000000, -3.250000000000000444 ) ) ;
#5669=CARTESIAN_POINT ( 'NONE',  ( -3.250000000000001776, 111.5625000000000000, -1.346194077712558279 ) ) ;
#5678=CARTESIAN_POINT ( 'NONE',  ( 1.990051048614449116E-16, 111.1249999972688158, 3.250000000000000444 ) ) ;
#5688=CARTESIAN_POINT ( 'NONE',  ( 1.658621287961228566E-16, 110.5624999986344079, 2.708734125000000326 ) ) ;
#5693=ORIENTED_EDGE ( 'NONE', *, *, #4907, .F. ) ;
#5697=ORIENTED_EDGE ( 'NONE', *, *, #5561, .T. ) ;
#5699=FACE_OUTER_BOUND ( 'NONE', #2268, .T. ) ;
#5708=CARTESIAN_POINT ( 'NONE',  ( 1.121994411437819084, 110.7499999986343937, 2.708734124999999882 ) ) ;
#5713=ORIENTED_EDGE ( 'NONE', *, *, #6076, .T. ) ;
#5727=LINE ( 'NONE', #6651, #12020 ) ;
#5732=CARTESIAN_POINT ( 'NONE',  ( -1.915364268218909150, 110.6874999986344079, 1.915364268218909594 ) ) ;
#5740=CARTESIAN_POINT ( 'NONE',  ( -2.298097038856279806, 111.4999999972688158, -2.298097038856279362 ) ) ;
#5750=CARTESIAN_POINT ( 'NONE',  ( -2.708734124999999882, 112.9999999986343937, 1.121994411437818862 ) ) ;
#5751=CARTESIAN_POINT ( 'NONE',  ( 3.249999999999999556, 112.8124999972688158, -1.346194077712561610 ) ) ;
#5753=VERTEX_POINT ( 'NONE', #12096 ) ;
#5765=CARTESIAN_POINT ( 'NONE',  ( -2.708734125000000326, 114.1249999986344079, -1.121994411437818195 ) ) ;
#5766=CARTESIAN_POINT ( 'NONE',  ( 1.990051048614449116E-16, 112.2500000000000000, 3.250000000000000444 ) ) ;
#5792=FACE_OUTER_BOUND ( 'NONE', #7251, .T. ) ;
#5806=LINE ( 'NONE', #4736, #2424 ) ;
#5809=CARTESIAN_POINT ( 'NONE',  ( -2.708734125000000770, 113.8749999986343937, -1.121994411437818639 ) ) ;
#5810=CARTESIAN_POINT ( 'NONE',  ( -5.970153145843347347E-16, 112.6249999972688158, -3.250000000000000444 ) ) ;
#5813=EDGE_LOOP ( 'NONE', ( #7963, #3972, #5914, #4566 ) ) ;
#5820=DIRECTION ( 'NONE',  ( -0.000000000000000000, -1.000000000000000000, -0.000000000000000000 ) ) ;
#5822=EDGE_CURVE ( 'NONE', #2754, #1921, #5912, .T. ) ;
#5825=CARTESIAN_POINT ( 'NONE',  ( -5.970153145843347347E-16, 114.6249999972688158, -3.250000000000000444 ) ) ;
#5826=DIRECTION ( 'NONE',  ( -0.000000000000000000, -1.000000000000000000, -0.000000000000000000 ) ) ;
#5827=CARTESIAN_POINT ( 'NONE',  ( 1.121994411437819084, 114.3749999986344221, -2.708734124999999437 ) ) ;
#5829=VERTEX_POINT ( 'NONE', #4785 ) ;
#5831=ORIENTED_EDGE ( 'NONE', *, *, #4726, .T. ) ;
#5839=CARTESIAN_POINT ( 'NONE',  ( -1.121994411437820194, 110.9999999986343937, -2.708734124999999882 ) ) ;
#5846=DIRECTION ( 'NONE',  ( 0.000000000000000000, 1.000000000000000000, 0.000000000000000000 ) ) ;
#5857=ORIENTED_EDGE ( 'NONE', *, *, #4576, .T. ) ;
#5867=EDGE_CURVE ( 'NONE', #3256, #12241, #12314, .T. ) ;
#5871=CARTESIAN_POINT ( 'NONE',  ( 1.658621287961228566E-16, 111.5624999986344079, 2.708734125000000326 ) ) ;
#5875=DIRECTION ( 'NONE',  ( -0.000000000000000000, 1.000000000000000000, -0.000000000000000000 ) ) ;
#5885=CARTESIAN_POINT ( 'NONE',  ( 0.000000000000000000, 165.0000000000000000, 0.000000000000000000 ) ) ;
#5886=CARTESIAN_POINT ( 'NONE',  ( 2.571758278209439492E-16, 153.0000000000000000, -2.099999999999998312 ) ) ;
#5890=CARTESIAN_POINT ( 'NONE',  ( 2.708734124999999882, 113.5624999986344079, 0.000000000000000000 ) ) ;
#5900=CARTESIAN_POINT ( 'NONE',  ( 1.915364268218908927, 111.1874999986344079, -1.915364268218909816 ) ) ;
#5909=CARTESIAN_POINT ( 'NONE',  ( 2.708734124999999882, 110.4374999986344079, 0.000000000000000000 ) ) ;
#5912=LINE ( 'NONE', #3853, #7463 ) ;
#5914=ORIENTED_EDGE ( 'NONE', *, *, #2691, .T. ) ;
#5923=CARTESIAN_POINT ( 'NONE',  ( -1.346194077712560944, 111.1874999972687874, 3.249999999999998668 ) ) ;
#5929=CARTESIAN_POINT ( 'NONE',  ( 2.708734125000000326, 112.3124999986344079, 0.000000000000000000 ) ) ;
#5946=CARTESIAN_POINT ( 'NONE',  ( -4.975863863883684959E-16, 112.3124999986344079, -2.708734124999999882 ) ) ;
#5971=EDGE_CURVE ( 'NONE', #1174, #3450, #10888, .T. ) ;
#5987=CARTESIAN_POINT ( 'NONE',  ( -8.000000000000000000, 115.0000000000000000, -5.999999999999998224 ) ) ;
#5990=CARTESIAN_POINT ( 'NONE',  ( -2.708734125000000770, 112.8749999986344079, -1.121994411437818639 ) ) ;
#5991=CARTESIAN_POINT ( 'NONE',  ( 3.250000000000000444, 113.9374999972688158, 1.346194077712559389 ) ) ;
#6009=CARTESIAN_POINT ( 'NONE',  ( -2.708734125000000326, 113.1249999986344079, -1.121994411437818195 ) ) ;
#6021=VECTOR ( 'NONE', #10441, 1000.000000000000000 ) ;
#6027=SURFACE_STYLE_USAGE ( .BOTH. , #2220 ) ;
#6034=CARTESIAN_POINT ( 'NONE',  ( 2.708734125000000326, 113.3749999986344079, 1.121994411437818862 ) ) ;
#6048=DIRECTION ( 'NONE',  ( 0.000000000000000000, 0.000000000000000000, 1.000000000000000000 ) ) ;
#6050=CARTESIAN_POINT ( 'NONE',  ( -2.708734125000000326, 111.7499999986344079, 1.121994411437818862 ) ) ;
#6052=AXIS2_PLACEMENT_3D ( 'NONE', #3806, #10530, #947 ) ;
#6076=EDGE_CURVE ( 'NONE', #8201, #2754, #8471, .T. ) ;
#6077=STYLED_ITEM ( 'NONE', ( #9812 ), #589 ) ;
#6089=( NAMED_UNIT ( * ) SI_UNIT ( $, .STERADIAN. ) SOLID_ANGLE_UNIT ( ) );
#6092=DIRECTION ( 'NONE',  ( 0.000000000000000000, 0.000000000000000000, 1.000000000000000000 ) ) ;
#6098=CARTESIAN_POINT ( 'NONE',  ( 1.915364268218909594, 112.4374999986344079, 1.915364268218909594 ) ) ;
#6141=CARTESIAN_POINT ( 'NONE',  ( 2.708734124999999882, 114.2499999986344079, -1.121994411437820416 ) ) ;
#6144=( NAMED_UNIT ( * ) PLANE_ANGLE_UNIT ( ) SI_UNIT ( $, .RADIAN. ) );
#6153=CARTESIAN_POINT ( 'NONE',  ( 1.915364268218909594, 113.4374999986344079, 1.915364268218909594 ) ) ;
#6162=CARTESIAN_POINT ( 'NONE',  ( 3.250000000000000444, 113.8749999972688158, 0.000000000000000000 ) ) ;
#6186=CARTESIAN_POINT ( 'NONE',  ( 1.121994411437818862, 110.7499999986343937, 2.708734124999999882 ) ) ;
#6187=CIRCLE ( 'NONE', #3967, 9.999999999999998224 ) ;
#6202=CARTESIAN_POINT ( 'NONE',  ( 1.346194077712585591, 114.6874999972688158, -3.249999999999974687 ) ) ;
#6219=CARTESIAN_POINT ( 'NONE',  ( -1.121994411437818862, 112.6249999986343937, 2.708734125000000326 ) ) ;
#6231=DIRECTION ( 'NONE',  ( 0.000000000000000000, 1.000000000000000000, 0.000000000000000000 ) ) ;
#6239=CARTESIAN_POINT ( 'NONE',  ( 0.000000000000000000, 153.0000000000000000, 0.000000000000000000 ) ) ;
#6245=ADVANCED_FACE ( 'NONE', ( #8984 ), #7188, .T. ) ;
#6251=CARTESIAN_POINT ( 'NONE',  ( 3.250000000000000444, 112.0000000000000000, 0.000000000000000000 ) ) ;
#6260=CARTESIAN_POINT ( 'NONE',  ( -5.970153145843347347E-16, 110.7500000000000000, -3.250000000000000444 ) ) ;
#6263=CARTESIAN_POINT ( 'NONE',  ( 1.121994411437819084, 111.4999999986343937, 2.708734125000000326 ) ) ;
#6270=CARTESIAN_POINT ( 'NONE',  ( 1.990051048614449116E-16, 111.2500000000000000, 3.250000000000000444 ) ) ;
#6271=LINE ( 'NONE', #1229, #4059 ) ;
#6278=CARTESIAN_POINT ( 'NONE',  ( 1.346194077712559389, 110.1875000000000142, 3.250000000000000444 ) ) ;
#6282=CARTESIAN_POINT ( 'NONE',  ( -5.970153145843347347E-16, 113.7500000000000000, -3.250000000000000444 ) ) ;
#6283=ADVANCED_FACE ( 'NONE', ( #9165 ), #12058, .T. ) ;
#6306=ORIENTED_EDGE ( 'NONE', *, *, #1256, .F. ) ;
#6325=CARTESIAN_POINT ( 'NONE',  ( -1.121994411437819084, 112.6249999986343937, 2.708734125000000326 ) ) ;
#6326=CARTESIAN_POINT ( 'NONE',  ( -2.708734125000000326, 113.1249999986343937, -1.121994411437818195 ) ) ;
#6334=DIRECTION ( 'NONE',  ( 0.000000000000000000, 0.000000000000000000, -1.000000000000000000 ) ) ;
#6340=CARTESIAN_POINT ( 'NONE',  ( 1.346194077712564940, 111.6874999972687732, -3.249999999999993783 ) ) ;
#6341=CARTESIAN_POINT ( 'NONE',  ( 2.298097038856279806, 113.1250000000000000, 2.298097038856279806 ) ) ;
#6344=CARTESIAN_POINT ( 'NONE',  ( -5.970153145843347347E-16, 112.6249999972688158, -3.250000000000000444 ) ) ;
#6351=VERTEX_POINT ( 'NONE', #10484 ) ;
#6371=CARTESIAN_POINT ( 'NONE',  ( 3.250000000000000444, 110.9374999972688016, 1.346194077712559167 ) ) ;
#6389=CARTESIAN_POINT ( 'NONE',  ( -1.121994411437820194, 112.2499999986344079, -2.708734124999999437 ) ) ;
#6405=CARTESIAN_POINT ( 'NONE',  ( -3.250000000000000444, 113.5000000000000000, 3.980102097228898231E-16 ) ) ;
#6410=CARTESIAN_POINT ( 'NONE',  ( 3.250000000000000444, 112.9374999972688016, 1.346194077712559167 ) ) ;
#6436=CARTESIAN_POINT ( 'NONE',  ( -1.121994411437820194, 112.2499999986344079, -2.708734124999999437 ) ) ;
#6444=CARTESIAN_POINT ( 'NONE',  ( -3.250000000000001776, 112.5625000000000000, -1.346194077712558279 ) ) ;
#6449=CARTESIAN_POINT ( 'NONE',  ( -2.708734124999999882, 111.9999999986343937, 1.121994411437818862 ) ) ;
#6465=ORIENTED_EDGE ( 'NONE', *, *, #7466, .F. ) ;
#6479=DIRECTION ( 'NONE',  ( -0.000000000000000000, -1.000000000000000000, -0.000000000000000000 ) ) ;
#6480=CIRCLE ( 'NONE', #5097, 9.999999999999998224 ) ;
#6502=CARTESIAN_POINT ( 'NONE',  ( 2.708734124999999882, 113.5624999986344079, 0.000000000000000000 ) ) ;
#6503=DIRECTION ( 'NONE',  ( -0.000000000000000000, 1.000000000000000000, -0.000000000000000000 ) ) ;
#6509=CARTESIAN_POINT ( 'NONE',  ( -2.298097038856279806, 112.6250000000000000, -2.298097038856279362 ) ) ;
#6512=ADVANCED_FACE ( 'NONE', ( #7971 ), #4471, .F. ) ;
#6515=CARTESIAN_POINT ( 'NONE',  ( 1.121994411437819084, 111.3749999986344221, -2.708734124999999437 ) ) ;
#6550=EDGE_CURVE ( 'NONE', #9788, #421, #1239, .T. ) ;
#6556=CARTESIAN_POINT ( 'NONE',  ( -1.915364268218908927, 111.9374999986344079, 1.915364268218909150 ) ) ;
#6568=AXIS2_PLACEMENT_3D ( 'NONE', #2922, #3041, #10581 ) ;
#6569=CARTESIAN_POINT ( 'NONE',  ( -1.915364268218909594, 111.1874999986344079, -1.915364268218908927 ) ) ;
#6574=ADVANCED_FACE ( 'NONE', ( #3439 ), #1502, .T. ) ;
#6616=CARTESIAN_POINT ( 'NONE',  ( -1.915364268218909594, 114.1874999986344079, -1.915364268218908927 ) ) ;
#6617=CARTESIAN_POINT ( 'NONE',  ( 3.250000000000000444, 112.9374999972688016, 1.346194077712559389 ) ) ;
#6631=DIRECTION ( 'NONE',  ( -0.000000000000000000, 1.000000000000000000, -0.000000000000000000 ) ) ;
#6643=( BOUNDED_CURVE ( )  B_SPLINE_CURVE ( 2, ( #8671, #133, #1263, #4947, #3948, #7743, #8793, #4007, #11557 ),
 .UNSPECIFIED., .F., .F. ) 
 B_SPLINE_CURVE_WITH_KNOTS ( ( 3, 2, 2, 2, 3 ),
 ( 0.06250000000000005551, 0.09375000000000008327, 0.1250000000000001110, 0.1562500000000001388, 0.1875000000000001665 ),
 .UNSPECIFIED. ) 
 CURVE ( )  GEOMETRIC_REPRESENTATION_ITEM ( )  RATIONAL_B_SPLINE_CURVE ( ( 0.9999999999999998890, 0.9238795325112868495, 1.000000000000000000, 0.9238795325112867385, 1.000000000000000000, 0.9238795325112867385, 1.000000000000000000, 0.9238795325112862944, 1.000000000000000444 ) ) 
 REPRESENTATION_ITEM ( '' )  );
#6651=CARTESIAN_POINT ( 'NONE',  ( 3.980102097228898231E-16, 110.0000000000000000, -3.250000000000000444 ) ) ;
#6659=CARTESIAN_POINT ( 'NONE',  ( 2.708734125000000326, 110.3124999986344079, 0.000000000000000000 ) ) ;
#6662=EDGE_CURVE ( 'NONE', #5753, #5494, #1806, .T. ) ;
#6663=( BOUNDED_CURVE ( )  B_SPLINE_CURVE ( 2, ( #6344, #8326, #859, #1547, #10260, #6410, #11276, #10197, #1733 ),
 .UNSPECIFIED., .F., .F. ) 
 B_SPLINE_CURVE_WITH_KNOTS ( ( 3, 2, 2, 2, 3 ),
 ( 0.4375000000000003886, 0.4687500000000003886, 0.5000000000000004441, 0.5312500000000004441, 0.5625000000000004441 ),
 .UNSPECIFIED. ) 
 CURVE ( )  GEOMETRIC_REPRESENTATION_ITEM ( )  RATIONAL_B_SPLINE_CURVE ( ( 0.9999999999999990008, 0.9238795325112877377, 1.000000000000000000, 0.9238795325112867385, 1.000000000000000000, 0.9238795325112867385, 1.000000000000000000, 0.9238795325112856283, 1.000000000000001110 ) ) 
 REPRESENTATION_ITEM ( '' )  );
#6678=CARTESIAN_POINT ( 'NONE',  ( 2.708734124999999437, 112.4999999986344079, -1.121994411437820638 ) ) ;
#6679=CARTESIAN_POINT ( 'NONE',  ( -3.250000000000000444, 111.3124999972687874, 1.346194077712559389 ) ) ;
#6681=PRODUCT_DEFINITION_SHAPE ( 'NONE', 'NONE',  #5048 ) ;
#6682=ADVANCED_FACE ( 'NONE', ( #1627 ), #10212, .T. ) ;
#6696=CARTESIAN_POINT ( 'NONE',  ( -1.346194077712559389, 113.3125000000000142, 3.250000000000000444 ) ) ;
#6698=CARTESIAN_POINT ( 'NONE',  ( -4.975863863883684959E-16, 114.3124999986344079, -2.708734124999999882 ) ) ;
#6709=LINE ( 'NONE', #9560, #6021 ) ;
#6711=AXIS2_PLACEMENT_3D ( 'NONE', #4366, #12174, #3446 ) ;
#6722=EDGE_LOOP ( 'NONE', ( #7835, #494, #11465, #7561 ) ) ;
#6740=CARTESIAN_POINT ( 'NONE',  ( -2.708734125000000326, 110.8124999986344079, 3.317242575922457132E-16 ) ) ;
#6741=CARTESIAN_POINT ( 'NONE',  ( 1.346194077712559833, 111.6874999972688016, -3.250000000000000000 ) ) ;
#6748=CYLINDRICAL_SURFACE ( 'NONE', #11872, 2.099999999999993427 ) ;
#6754=CARTESIAN_POINT ( 'NONE',  ( 2.979367062500000163, 114.1562499993171969, 0.000000000000000000 ) ) ;
#6755=CARTESIAN_POINT ( 'NONE',  ( -1.121994411437819084, 112.8749999986344079, 2.708734124999999882 ) ) ;
#6765=CARTESIAN_POINT ( 'NONE',  ( -2.708734125000000770, 110.8749999986343937, -1.121994411437818639 ) ) ;
#6776=CARTESIAN_POINT ( 'NONE',  ( 2.298097038856278918, 112.8750000000000000, -2.298097038856279806 ) ) ;
#6784=CARTESIAN_POINT ( 'NONE',  ( -5.970153145843347347E-16, 113.6249999972688158, -3.250000000000000444 ) ) ;
#6802=VERTEX_POINT ( 'NONE', #8584 ) ;
#6803=CARTESIAN_POINT ( 'NONE',  ( 1.915364268218908927, 112.1874999986344079, -1.915364268218909816 ) ) ;
#6804=CARTESIAN_POINT ( 'NONE',  ( 2.298097038856279806, 110.9999999972688158, 2.298097038856279806 ) ) ;
#6807=ORIENTED_EDGE ( 'NONE', *, *, #3057, .T. ) ;
#6812=DIRECTION ( 'NONE',  ( 0.000000000000000000, 0.000000000000000000, 1.000000000000000000 ) ) ;
#6818=DIRECTION ( 'NONE',  ( 0.000000000000000000, 0.000000000000000000, 1.000000000000000000 ) ) ;
#6820=CARTESIAN_POINT ( 'NONE',  ( -2.708734124999999882, 112.9999999986344079, 1.121994411437819084 ) ) ;
#6828=CARTESIAN_POINT ( 'NONE',  ( -5.970153145843347347E-16, 112.6249999972688158, -3.250000000000000444 ) ) ;
#6847=CARTESIAN_POINT ( 'NONE',  ( -1.346194077712542736, 113.5624999972688016, -3.250000000000017764 ) ) ;
#6855=ORIENTED_EDGE ( 'NONE', *, *, #11291, .T. ) ;
#6856=DIRECTION ( 'NONE',  ( 0.000000000000000000, -1.000000000000000000, 0.000000000000000000 ) ) ;
#6865=CARTESIAN_POINT ( 'NONE',  ( 1.121994411437819528, 111.1249999986343937, -2.708734124999999882 ) ) ;
#6866=CARTESIAN_POINT ( 'NONE',  ( -1.346194077712559389, 112.1874999972688016, 3.250000000000000444 ) ) ;
#6880=CARTESIAN_POINT ( 'NONE',  ( 0.000000000000000000, 110.0000000000000000, 0.000000000000000000 ) ) ;
#6881=CARTESIAN_POINT ( 'NONE',  ( 1.915364268218908705, 114.4374999986344079, -1.915364268218909594 ) ) ;
#6900=( NAMED_UNIT ( * ) SI_UNIT ( $, .STERADIAN. ) SOLID_ANGLE_UNIT ( ) );
#6908=DIRECTION ( 'NONE',  ( -0.000000000000000000, 1.000000000000000000, -0.000000000000000000 ) ) ;
#6924=CARTESIAN_POINT ( 'NONE',  ( 1.915364268218909594, 112.4374999986344079, 1.915364268218909594 ) ) ;
#6925=CARTESIAN_POINT ( 'NONE',  ( 2.298097038856278918, 113.7499999972688158, -2.298097038856279806 ) ) ;
#6934=VECTOR ( 'NONE', #2987, 1000.000000000000000 ) ;
#6936=CYLINDRICAL_SURFACE ( 'NONE', #5486, 9.999999999999998224 ) ;
#6957=VECTOR ( 'NONE', #7252, 1000.000000000000000 ) ;
#6964=CARTESIAN_POINT ( 'NONE',  ( 1.915364268218908927, 113.1874999986344079, -1.915364268218909816 ) ) ;
#6980=CARTESIAN_POINT ( 'NONE',  ( -1.915364268218909150, 113.6874999986344079, 1.915364268218909594 ) ) ;
#6992=ORIENTED_EDGE ( 'NONE', *, *, #5971, .T. ) ;
#7001=EDGE_CURVE ( 'NONE', #861, #9973, #4161, .T. ) ;
#7007=PRODUCT_DEFINITION_CONTEXT ( 'detailed design', #2548, 'design' ) ;
#7011=DIRECTION ( 'NONE',  ( -0.000000000000000000, -1.000000000000000000, -0.000000000000000000 ) ) ;
#7020=( LENGTH_UNIT ( ) NAMED_UNIT ( * ) SI_UNIT ( .MILLI., .METRE. ) );
#7025=CARTESIAN_POINT ( 'NONE',  ( -2.708734125000000770, 112.8749999986344079, -1.121994411437818639 ) ) ;
#7027=ORIENTED_EDGE ( 'NONE', *, *, #9513, .F. ) ;
#7047=CARTESIAN_POINT ( 'NONE',  ( 2.708734125000000326, 114.3124999986344079, 0.000000000000000000 ) ) ;
#7066=DIRECTION ( 'NONE',  ( -0.000000000000000000, 1.000000000000000000, -0.000000000000000000 ) ) ;
#7072=CARTESIAN_POINT ( 'NONE',  ( 1.990051048614449116E-16, 112.1249999972688158, 3.250000000000000444 ) ) ;
#7074=CARTESIAN_POINT ( 'NONE',  ( -2.708734125000000770, 111.8749999986343937, -1.121994411437818639 ) ) ;
#7088=CARTESIAN_POINT ( 'NONE',  ( 3.250000000000000444, 114.8749999972688158, 0.000000000000000000 ) ) ;
#7092=CARTESIAN_POINT ( 'NONE',  ( 1.121994411437819528, 111.1249999986343937, -2.708734124999999882 ) ) ;
#7095=DIRECTION ( 'NONE',  ( 0.000000000000000000, 1.000000000000000000, 0.000000000000000000 ) ) ;
#7099=DIRECTION ( 'NONE',  ( 0.000000000000000000, 0.000000000000000000, -1.000000000000000000 ) ) ;
#7104=FACE_OUTER_BOUND ( 'NONE', #1676, .T. ) ;
#7106=CARTESIAN_POINT ( 'NONE',  ( -2.298097038856279362, 113.3750000000000000, 2.298097038856279806 ) ) ;
#7121=FACE_OUTER_BOUND ( 'NONE', #5084, .T. ) ;
#7128=CARTESIAN_POINT ( 'NONE',  ( 1.346194077712550063, 111.1874999999999858, 3.250000000000008438 ) ) ;
#7134=CARTESIAN_POINT ( 'NONE',  ( 2.708734124999999882, 113.2499999986344079, -1.121994411437820416 ) ) ;
#7136=SHAPE_REPRESENTATION ( 'Central Drive Shaft Post', ( #1612 ), #9157 ) ;
#7137=VERTEX_POINT ( 'NONE', #8450 ) ;
#7150=CARTESIAN_POINT ( 'NONE',  ( 1.658621287961228566E-16, 111.5624999986344079, 2.708734125000000326 ) ) ;
#7157=ORIENTED_EDGE ( 'NONE', *, *, #5867, .F. ) ;
#7162=FACE_OUTER_BOUND ( 'NONE', #126, .T. ) ;
#7170=CARTESIAN_POINT ( 'NONE',  ( 1.990051048614449116E-16, 112.1249999972688158, 3.250000000000000444 ) ) ;
#7183=CARTESIAN_POINT ( 'NONE',  ( 3.249999999999999556, 111.9375000000000000, -1.346194077712561166 ) ) ;
#7188=CYLINDRICAL_SURFACE ( 'NONE', #11043, 3.250000000000000444 ) ;
#7202=ADVANCED_BREP_SHAPE_REPRESENTATION ( '', ( #589, #1612 ), #9157 ) ;
#7213=CARTESIAN_POINT ( 'NONE',  ( 2.708734125000000326, 114.3124999986344079, 0.000000000000000000 ) ) ;
#7215=CARTESIAN_POINT ( 'NONE',  ( 2.708734124999999882, 110.5624999986344079, 0.000000000000000000 ) ) ;
#7216=DIRECTION ( 'NONE',  ( 0.000000000000000000, -0.000000000000000000, 1.000000000000000000 ) ) ;
#7251=EDGE_LOOP ( 'NONE', ( #5302, #4126, #2335, #359 ) ) ;
#7252=DIRECTION ( 'NONE',  ( -0.000000000000000000, -1.000000000000000000, -0.000000000000000000 ) ) ;
#7262=CARTESIAN_POINT ( 'NONE',  ( -1.121994411437819084, 113.6249999986344079, 2.708734125000000326 ) ) ;
#7306=ORIENTED_EDGE ( 'NONE', *, *, #153, .T. ) ;
#7312=CARTESIAN_POINT ( 'NONE',  ( 1.990051048614449116E-16, 112.2500000000000000, 3.250000000000000444 ) ) ;
#7315=EDGE_CURVE ( 'NONE', #10309, #12150, #5727, .T. ) ;
#7319=CARTESIAN_POINT ( 'NONE',  ( 0.000000000000000000, 110.0000000000000000, 0.000000000000000000 ) ) ;
#7323=ORIENTED_EDGE ( 'NONE', *, *, #8878, .T. ) ;
#7326=CARTESIAN_POINT ( 'NONE',  ( 1.915364268218908927, 114.1874999986344079, -1.915364268218909816 ) ) ;
#7327=CARTESIAN_POINT ( 'NONE',  ( 1.121994411437819084, 113.3749999986344079, -2.708734124999999437 ) ) ;
#7332=DIRECTION ( 'NONE',  ( 0.000000000000000000, 0.000000000000000000, 1.000000000000000000 ) ) ;
#7339=CARTESIAN_POINT ( 'NONE',  ( 3.250000000000000444, 111.9374999972688016, 1.346194077712559167 ) ) ;
#7341=CARTESIAN_POINT ( 'NONE',  ( 1.346194077712559389, 112.1875000000000142, 3.250000000000000444 ) ) ;
#7346=ORIENTED_EDGE ( 'NONE', *, *, #9657, .T. ) ;
#7348=DIRECTION ( 'NONE',  ( 0.000000000000000000, 0.000000000000000000, 1.000000000000000000 ) ) ;
#7358=AXIS2_PLACEMENT_3D ( 'NONE', #2018, #5826, #9728 ) ;
#7372=CARTESIAN_POINT ( 'NONE',  ( -1.121994411437820194, 113.2499999986344079, -2.708734124999999437 ) ) ;
#7389=CARTESIAN_POINT ( 'NONE',  ( 1.915364268218909150, 112.6874999986344079, 1.915364268218909150 ) ) ;
#7402=CARTESIAN_POINT ( 'NONE',  ( 1.990051048614449116E-16, 114.1249999972688158, 3.250000000000000444 ) ) ;
#7405=CARTESIAN_POINT ( 'NONE',  ( 2.298097038856279806, 111.1250000000000000, 2.298097038856279806 ) ) ;
#7414=EDGE_LOOP ( 'NONE', ( #5065, #4377, #11162, #5713, #245, #7346, #7639, #3918, #1267, #8752, #8914, #1764 ) ) ;
#7425=ORIENTED_EDGE ( 'NONE', *, *, #1152, .F. ) ;
#7435=CARTESIAN_POINT ( 'NONE',  ( 1.915364268218908705, 112.4374999986344079, -1.915364268218909594 ) ) ;
#7437=CARTESIAN_POINT ( 'NONE',  ( 3.249999999999999556, 113.9375000000000000, -1.346194077712561166 ) ) ;
#7448=CARTESIAN_POINT ( 'NONE',  ( 2.708734124999999437, 112.4999999986344079, -1.121994411437820638 ) ) ;
#7449=CARTESIAN_POINT ( 'NONE',  ( 2.708734124999999437, 111.4999999986343937, -1.121994411437820416 ) ) ;
#7463=VECTOR ( 'NONE', #4040, 1000.000000000000000 ) ;
#7466=EDGE_CURVE ( 'NONE', #421, #5123, #6271, .T. ) ;
#7493=CARTESIAN_POINT ( 'NONE',  ( 1.915364268218909594, 110.4374999986344079, 1.915364268218909594 ) ) ;
#7502=CARTESIAN_POINT ( 'NONE',  ( 3.250000000000000444, 110.0000000000000000, 0.000000000000000000 ) ) ;
#7507=CARTESIAN_POINT ( 'NONE',  ( -2.708734125000000326, 111.1249999986343937, -1.121994411437818195 ) ) ;
#7537=CARTESIAN_POINT ( 'NONE',  ( 3.250000000000000444, 110.8749999972688158, 0.000000000000000000 ) ) ;
#7543=CARTESIAN_POINT ( 'NONE',  ( -1.346194077712555837, 111.5624999972688158, -3.250000000000004885 ) ) ;
#7551=CARTESIAN_POINT ( 'NONE',  ( 1.915364268218909150, 113.6874999986344079, 1.915364268218909150 ) ) ;
#7555=ORIENTED_EDGE ( 'NONE', *, *, #2351, .T. ) ;
#7561=ORIENTED_EDGE ( 'NONE', *, *, #2351, .F. ) ;
#7564=VECTOR ( 'NONE', #622, 1000.000000000000000 ) ;
#7570=AXIS2_PLACEMENT_3D ( 'NONE', #4223, #5349, #4285 ) ;
#7580=COLOUR_RGB ( '', 0.40784314, 0.44705882, 0.49803922) ;
#7592=FACE_OUTER_BOUND ( 'NONE', #4625, .T. ) ;
#7595=CARTESIAN_POINT ( 'NONE',  ( 2.979367062500000163, 110.7187499979516190, 0.000000000000000000 ) ) ;
#7599=CARTESIAN_POINT ( 'NONE',  ( 2.708734124999999882, 114.4374999986344079, 0.000000000000000000 ) ) ;
#7612=CARTESIAN_POINT ( 'NONE',  ( -2.708734125000000326, 111.1249999986343937, -1.121994411437818195 ) ) ;
#7613=CARTESIAN_POINT ( 'NONE',  ( -2.298097038856279362, 113.2499999972688158, 2.298097038856279806 ) ) ;
#7615=ORIENTED_EDGE ( 'NONE', *, *, #5382, .T. ) ;
#7627=FACE_OUTER_BOUND ( 'NONE', #4017, .T. ) ;
#7628=CARTESIAN_POINT ( 'NONE',  ( 1.121994411437819084, 111.7499999986343795, 2.708734124999999882 ) ) ;
#7639=ORIENTED_EDGE ( 'NONE', *, *, #11976, .T. ) ;
#7653=CARTESIAN_POINT ( 'NONE',  ( -3.250000000000000444, 111.4375000000000000, 1.346194077712559167 ) ) ;
#7654=CARTESIAN_POINT ( 'NONE',  ( -2.708734125000000326, 110.7499999986343937, 1.121994411437818862 ) ) ;
#7671=CARTESIAN_POINT ( 'NONE',  ( -1.121994411437820416, 110.9999999986343937, -2.708734124999999882 ) ) ;
#7682=VERTEX_POINT ( 'NONE', #4704 ) ;
#7688=CARTESIAN_POINT ( 'NONE',  ( -1.346194077712559389, 112.3125000000000000, 3.250000000000000444 ) ) ;
#7706=FILL_AREA_STYLE ('',( #8627 ) ) ;
#7735=CARTESIAN_POINT ( 'NONE',  ( 1.121994411437818862, 113.4999999986344079, 2.708734125000000326 ) ) ;
#7736=CARTESIAN_POINT ( 'NONE',  ( -2.298097038856279806, 112.4999999972688158, -2.298097038856279362 ) ) ;
#7737=ORIENTED_EDGE ( 'NONE', *, *, #9181, .T. ) ;
#7743=CARTESIAN_POINT ( 'NONE',  ( -3.250000000000001776, 110.5625000000000000, -1.346194077712558279 ) ) ;
#7748=CYLINDRICAL_SURFACE ( 'NONE', #11151, 3.250000000000000444 ) ;
#7770=DIRECTION ( 'NONE',  ( -0.000000000000000000, 1.000000000000000000, -0.000000000000000000 ) ) ;
#7773=CARTESIAN_POINT ( 'NONE',  ( -2.298097038856279806, 111.6250000000000000, -2.298097038856279362 ) ) ;
#7779=AXIS2_PLACEMENT_3D ( 'NONE', #704, #11362, #4436 ) ;
#7814=CARTESIAN_POINT ( 'NONE',  ( 1.658621287961228320E-16, 113.8124999986344079, 2.708734124999999882 ) ) ;
#7822=CARTESIAN_POINT ( 'NONE',  ( 2.708734125000000326, 110.3749999986344079, 1.121994411437819084 ) ) ;
#7823=DIRECTION ( 'NONE',  ( 0.000000000000000000, 0.000000000000000000, 1.000000000000000000 ) ) ;
#7833=CARTESIAN_POINT ( 'NONE',  ( -5.970153145843347347E-16, 111.7500000000000000, -3.250000000000000444 ) ) ;
#7835=ORIENTED_EDGE ( 'NONE', *, *, #9592, .F. ) ;
#7849=CARTESIAN_POINT ( 'NONE',  ( 1.121994411437819528, 112.1249999986343937, -2.708734124999999882 ) ) ;
#7851=CARTESIAN_POINT ( 'NONE',  ( 1.990051048614449116E-16, 111.1249999972688158, 3.250000000000000444 ) ) ;
#7860=ORIENTED_EDGE ( 'NONE', *, *, #9421, .T. ) ;
#7868=CARTESIAN_POINT ( 'NONE',  ( -1.121994411437819084, 111.8749999986343937, 2.708734124999999882 ) ) ;
#7882=VERTEX_POINT ( 'NONE', #1463 ) ;
#7890=CARTESIAN_POINT ( 'NONE',  ( 1.915364268218909594, 111.4374999986344079, 1.915364268218909594 ) ) ;
#7892=EDGE_LOOP ( 'NONE', ( #8331, #10410, #7555, #8159 ) ) ;
#7903=( BOUNDED_CURVE ( )  B_SPLINE_CURVE ( 2, ( #7537, #6371, #5504, #10159, #4500 ),
 .UNSPECIFIED., .F., .F. ) 
 B_SPLINE_CURVE_WITH_KNOTS ( ( 3, 2, 3 ),
 ( 0.000000000000000000, 0.03125000000000002776, 0.06250000000000005551 ),
 .UNSPECIFIED. ) 
 CURVE ( )  GEOMETRIC_REPRESENTATION_ITEM ( )  RATIONAL_B_SPLINE_CURVE ( ( 1.000000000000000000, 0.9238795325112867385, 1.000000000000000000, 0.9238795325112866275, 1.000000000000000222 ) ) 
 REPRESENTATION_ITEM ( '' )  );
#7907=CARTESIAN_POINT ( 'NONE',  ( 2.708734125000000326, 113.3124999986344079, 0.000000000000000000 ) ) ;
#7912=DIRECTION ( 'NONE',  ( -0.000000000000000000, 1.000000000000000000, -0.000000000000000000 ) ) ;
#7917=ADVANCED_FACE ( 'NONE', ( #11756 ), #9927, .T. ) ;
#7933=CARTESIAN_POINT ( 'NONE',  ( -2.298097038856279806, 112.4999999972688158, -2.298097038856279362 ) ) ;
#7936=VERTEX_POINT ( 'NONE', #2209 ) ;
#7948=CARTESIAN_POINT ( 'NONE',  ( -2.298097038856279362, 110.3750000000000000, 2.298097038856279806 ) ) ;
#7963=ORIENTED_EDGE ( 'NONE', *, *, #3169, .F. ) ;
#7971=FACE_OUTER_BOUND ( 'NONE', #5335, .T. ) ;
#7996=CARTESIAN_POINT ( 'NONE',  ( 1.915364268218908927, 112.1874999986344079, -1.915364268218909816 ) ) ;
#8000=( NAMED_UNIT ( * ) SI_UNIT ( $, .STERADIAN. ) SOLID_ANGLE_UNIT ( ) );
#8006=DIRECTION ( 'NONE',  ( 1.734723475976805517E-15, -1.000000000000000000, 0.000000000000000000 ) ) ;
#8012=CARTESIAN_POINT ( 'NONE',  ( -2.708734125000000326, 112.7499999986343937, 1.121994411437818862 ) ) ;
#8030=VERTEX_POINT ( 'NONE', #8243 ) ;
#8033=ORIENTED_EDGE ( 'NONE', *, *, #7315, .T. ) ;
#8054=EDGE_LOOP ( 'NONE', ( #10682, #10643, #5857, #10367 ) ) ;
#8057=DIRECTION ( 'NONE',  ( 0.000000000000000000, -1.000000000000000000, 0.000000000000000000 ) ) ;
#8058=CARTESIAN_POINT ( 'NONE',  ( 1.658621287961228566E-16, 111.5624999986344079, 2.708734125000000326 ) ) ;
#8077=CARTESIAN_POINT ( 'NONE',  ( 1.915364268218908927, 112.1874999986344079, -1.915364268218909816 ) ) ;
#8083=ORIENTED_EDGE ( 'NONE', *, *, #9181, .F. ) ;
#8106=VERTEX_POINT ( 'NONE', #2933 ) ;
#8119=CARTESIAN_POINT ( 'NONE',  ( -5.970153145843347347E-16, 114.6249999972688158, -3.250000000000000444 ) ) ;
#8135=CARTESIAN_POINT ( 'NONE',  ( 3.250000000000000444, 110.0000000000000000, 0.000000000000000000 ) ) ;
#8136=CARTESIAN_POINT ( 'NONE',  ( 1.121994411437819084, 111.3749999986344079, -2.708734124999999437 ) ) ;
#8151=CARTESIAN_POINT ( 'NONE',  ( -5.970153145843347347E-16, 113.7500000000000000, -3.250000000000000444 ) ) ;
#8154=CARTESIAN_POINT ( 'NONE',  ( -1.346194077712581150, 114.1874999972687874, 3.249999999999978240 ) ) ;
#8159=ORIENTED_EDGE ( 'NONE', *, *, #9813, .F. ) ;
#8182=CARTESIAN_POINT ( 'NONE',  ( 1.915364268218909594, 113.4374999986344079, 1.915364268218909594 ) ) ;
#8196=CARTESIAN_POINT ( 'NONE',  ( -3.250000000000000444, 111.4375000000000000, 1.346194077712559389 ) ) ;
#8201=VERTEX_POINT ( 'NONE', #3114 ) ;
#8203=ORIENTED_EDGE ( 'NONE', *, *, #3107, .F. ) ;
#8205=CARTESIAN_POINT ( 'NONE',  ( 2.298097038856278918, 113.7499999972688158, -2.298097038856279806 ) ) ;
#8243=CARTESIAN_POINT ( 'NONE',  ( 2.571758278209431110E-16, 165.0000000000000000, -2.099999999999988987 ) ) ;
#8246=CARTESIAN_POINT ( 'NONE',  ( 3.250000000000000444, 114.8749999972688158, 0.000000000000000000 ) ) ;
#8247=CARTESIAN_POINT ( 'NONE',  ( 1.658621287961228320E-16, 112.8124999986344079, 2.708734124999999882 ) ) ;
#8249=AXIS2_PLACEMENT_3D ( 'NONE', #360, #4228, #5233 ) ;
#8256=DIRECTION ( 'NONE',  ( 1.000000000000000000, 0.000000000000000000, 0.000000000000000000 ) ) ;
#8262=CARTESIAN_POINT ( 'NONE',  ( 3.250000000000000444, 112.0000000000000000, 0.000000000000000000 ) ) ;
#8279=CIRCLE ( 'NONE', #2720, 3.250000000000000444 ) ;
#8308=CARTESIAN_POINT ( 'NONE',  ( -1.915364268218908927, 112.9374999986344079, 1.915364268218909150 ) ) ;
#8321=CARTESIAN_POINT ( 'NONE',  ( -1.346194077712560944, 113.6875000000000000, -3.249999999999999556 ) ) ;
#8323=EDGE_CURVE ( 'NONE', #10309, #9788, #11770, .T. ) ;
#8326=CARTESIAN_POINT ( 'NONE',  ( 1.346194077712572934, 112.6874999972688158, -3.249999999999987121 ) ) ;
#8331=ORIENTED_EDGE ( 'NONE', *, *, #5561, .F. ) ;
#8351=CARTESIAN_POINT ( 'NONE',  ( 1.121994411437819084, 111.3749999986344221, -2.708734124999999437 ) ) ;
#8352=DIRECTION ( 'NONE',  ( 0.000000000000000000, -1.000000000000000000, 0.000000000000000000 ) ) ;
#8366=CARTESIAN_POINT ( 'NONE',  ( 1.915364268218909150, 113.6874999986344079, 1.915364268218909150 ) ) ;
#8383=CARTESIAN_POINT ( 'NONE',  ( -3.250000000000001776, 110.5625000000000000, -1.346194077712558723 ) ) ;
#8394=ORIENTED_EDGE ( 'NONE', *, *, #196, .F. ) ;
#8399=LINE ( 'NONE', #7595, #4772 ) ;
#8400=( BOUNDED_SURFACE ( )  B_SPLINE_SURFACE ( 1, 2, ( 
 ( #10857, #2377, #3382, #6186, #10983, #2447, #10040, #12177, #3685, #7612, #10480, #2748, #5508, #8351, #2629, #4741, #8532, #9528, #4558, #8414, #11421, #12298, #6556, #10346, #3627, #1168, #9404, #6436, #1817, #10224, #7435, #6678, #951, #2872, #10290, #887, #1942, #1700, #3811, #5750, #4681, #1010, #5628, #7372, #11239, #5566, #8473, #4620, #6502, #2687, #7551, #3745, #1758, #4809, #12114, #11361, #9343, #2812, #6616, #11174, #9287, #10411, #1874, #769, #829 ),
 ( #3566, #12239, #7493, #11304, #5688, #9471, #8596, #246, #6740, #2241, #5059, #7671, #308, #6865, #4058, #1252, #1194, #10719, #10534, #10660, #5871, #2179, #1314, #6050, #9653, #9778, #2127, #3121, #2998, #7849, #6803, #11669, #5929, #9712, #6924, #3996, #8839, #4873, #57, #8782, #2001, #5990, #4118, #9836, #4935, #4995, #1068, #3937, #7907, #3179, #11726, #7735, #8660, #122, #6980, #183, #10783, #5809, #1133, #11488, #9595, #2940, #3873, #11547, #10599 ) ),
 .UNSPECIFIED., .F., .F., .F. ) 
 B_SPLINE_SURFACE_WITH_KNOTS ( ( 2, 2 ),
 ( 3, 2, 2, 2, 2, 2, 2, 2, 2, 2, 2, 2, 2, 2, 2, 2, 2, 2, 2, 2, 2, 2, 2, 2, 2, 2, 2, 2, 2, 2, 2, 2, 3 ),
 ( 0.000000000000000000, 1.000000000000000000 ),
 ( 0.000000000000000000, 0.03125000000000000000, 0.06250000000000000000, 0.09375000000000000000, 0.1250000000000000000, 0.1562500000000000000, 0.1875000000000000000, 0.2187500000000000000, 0.2500000000000000000, 0.2812500000000000000, 0.3125000000000000000, 0.3437500000000000000, 0.3750000000000000000, 0.4062500000000000000, 0.4375000000000000000, 0.4687500000000000000, 0.5000000000000000000, 0.5312500000000000000, 0.5625000000000000000, 0.5937500000000000000, 0.6250000000000000000, 0.6562500000000000000, 0.6875000000000000000, 0.7187500000000000000, 0.7500000000000000000, 0.7812500000000000000, 0.8125000000000000000, 0.8437500000000000000, 0.8750000000000000000, 0.9062500000000000000, 0.9375000000000000000, 0.9687500000000000000, 1.000000000000000000 ),
 .UNSPECIFIED. ) 
 GEOMETRIC_REPRESENTATION_ITEM ( )  RATIONAL_B_SPLINE_SURFACE ( (
 ( 1.000000000000000000, 0.9238795325112867385, 1.000000000000000000, 0.9238795325112867385, 1.000000000000000000, 0.9238795325112867385, 1.000000000000000000, 0.9238795325112867385, 1.000000000000000000, 0.9238795325112867385, 1.000000000000000000, 0.9238795325112867385, 1.000000000000000000, 0.9238795325112867385, 1.000000000000000000, 0.9238795325112867385, 1.000000000000000000, 0.9238795325112867385, 1.000000000000000000, 0.9238795325112867385, 1.000000000000000000, 0.9238795325112867385, 1.000000000000000000, 0.9238795325112867385, 1.000000000000000000, 0.9238795325112867385, 1.000000000000000000, 0.9238795325112867385, 1.000000000000000000, 0.9238795325112867385, 1.000000000000000000, 0.9238795325112867385, 1.000000000000000000, 0.9238795325112867385, 1.000000000000000000, 0.9238795325112867385, 1.000000000000000000, 0.9238795325112867385, 1.000000000000000000, 0.9238795325112867385, 1.000000000000000000, 0.9238795325112867385, 1.000000000000000000, 0.9238795325112867385, 1.000000000000000000, 0.9238795325112867385, 1.000000000000000000, 0.9238795325112867385, 1.000000000000000000, 0.9238795325112867385, 1.000000000000000000, 0.9238795325112867385, 1.000000000000000000, 0.9238795325112867385, 1.000000000000000000, 0.9238795325112867385, 1.000000000000000000, 0.9238795325112867385, 1.000000000000000000, 0.9238795325112867385, 1.000000000000000000, 0.9238795325112867385, 1.000000000000000000, 0.9238795325112867385, 1.000000000000000000),
 ( 1.000000000000000000, 0.9238795325112867385, 1.000000000000000000, 0.9238795325112867385, 1.000000000000000000, 0.9238795325112867385, 1.000000000000000000, 0.9238795325112867385, 1.000000000000000000, 0.9238795325112867385, 1.000000000000000000, 0.9238795325112867385, 1.000000000000000000, 0.9238795325112867385, 1.000000000000000000, 0.9238795325112867385, 1.000000000000000000, 0.9238795325112867385, 1.000000000000000000, 0.9238795325112867385, 1.000000000000000000, 0.9238795325112867385, 1.000000000000000000, 0.9238795325112867385, 1.000000000000000000, 0.9238795325112867385, 1.000000000000000000, 0.9238795325112867385, 1.000000000000000000, 0.9238795325112867385, 1.000000000000000000, 0.9238795325112867385, 1.000000000000000000, 0.9238795325112867385, 1.000000000000000000, 0.9238795325112867385, 1.000000000000000000, 0.9238795325112867385, 1.000000000000000000, 0.9238795325112867385, 1.000000000000000000, 0.9238795325112867385, 1.000000000000000000, 0.9238795325112867385, 1.000000000000000000, 0.9238795325112867385, 1.000000000000000000, 0.9238795325112867385, 1.000000000000000000, 0.9238795325112867385, 1.000000000000000000, 0.9238795325112867385, 1.000000000000000000, 0.9238795325112867385, 1.000000000000000000, 0.9238795325112867385, 1.000000000000000000, 0.9238795325112867385, 1.000000000000000000, 0.9238795325112867385, 1.000000000000000000, 0.9238795325112867385, 1.000000000000000000, 0.9238795325112867385, 1.000000000000000000) ) ) 
 REPRESENTATION_ITEM ( '' )  SURFACE ( )  );
#8414=CARTESIAN_POINT ( 'NONE',  ( 1.121994411437818862, 111.7499999986344079, 2.708734124999999882 ) ) ;
#8415=VECTOR ( 'NONE', #10149, 1000.000000000000000 ) ;
#8417=ORIENTED_EDGE ( 'NONE', *, *, #6076, .F. ) ;
#8428=CARTESIAN_POINT ( 'NONE',  ( -2.708734124999999882, 114.0624999986344079, 3.317242575922456639E-16 ) ) ;
#8442=AXIS2_PLACEMENT_3D ( 'NONE', #363, #6231, #8955 ) ;
#8444=CIRCLE ( 'NONE', #8249, 2.099999999999988987 ) ;
#8450=CARTESIAN_POINT ( 'NONE',  ( 1.224646799147353059E-15, 165.0000000000000000, 9.999999999999998224 ) ) ;
#8465=AXIS2_PLACEMENT_3D ( 'NONE', #1323, #2248, #11923 ) ;
#8469=DIRECTION ( 'NONE',  ( 0.000000000000000000, 1.000000000000000000, 0.000000000000000000 ) ) ;
#8471=( BOUNDED_CURVE ( )  B_SPLINE_CURVE ( 2, ( #12018, #6340, #1603, #5410, #12085, #7339, #10800, #4375, #2260 ),
 .UNSPECIFIED., .F., .F. ) 
 B_SPLINE_CURVE_WITH_KNOTS ( ( 3, 2, 2, 2, 3 ),
 ( 0.1875000000000001665, 0.2187500000000001943, 0.2500000000000002220, 0.2812500000000002220, 0.3125000000000002776 ),
 .UNSPECIFIED. ) 
 CURVE ( )  GEOMETRIC_REPRESENTATION_ITEM ( )  RATIONAL_B_SPLINE_CURVE ( ( 0.9999999999999995559, 0.9238795325112871826, 1.000000000000000000, 0.9238795325112867385, 1.000000000000000000, 0.9238795325112867385, 1.000000000000000000, 0.9238795325112860723, 1.000000000000000666 ) ) 
 REPRESENTATION_ITEM ( '' )  );
#8473=CARTESIAN_POINT ( 'NONE',  ( 1.915364268218908705, 113.4374999986344079, -1.915364268218909594 ) ) ;
#8474=CARTESIAN_POINT ( 'NONE',  ( 3.250000000000000444, 114.0000000000000000, 0.000000000000000000 ) ) ;
#8481=CARTESIAN_POINT ( 'NONE',  ( 1.990051048614449116E-16, 112.2500000000000000, 3.250000000000000444 ) ) ;
#8486=CARTESIAN_POINT ( 'NONE',  ( -2.708734125000000326, 112.1249999986343937, -1.121994411437818195 ) ) ;
#8492=VERTEX_POINT ( 'NONE', #9940 ) ;
#8493=EDGE_CURVE ( 'NONE', #7936, #5440, #3108, .T. ) ;
#8532=CARTESIAN_POINT ( 'NONE',  ( 2.708734124999999882, 111.5624999986344079, 0.000000000000000000 ) ) ;
#8533=CARTESIAN_POINT ( 'NONE',  ( 2.298097038856279806, 112.9999999972688158, 2.298097038856279806 ) ) ;
#8552=CARTESIAN_POINT ( 'NONE',  ( -1.915364268218908927, 111.9374999986344079, 1.915364268218909150 ) ) ;
#8570=DIRECTION ( 'NONE',  ( -0.000000000000000000, 1.000000000000000000, -0.000000000000000000 ) ) ;
#8575=CARTESIAN_POINT ( 'NONE',  ( -1.346194077712568049, 111.3124999999999858, 3.249999999999991118 ) ) ;
#8584=CARTESIAN_POINT ( 'NONE',  ( 3.250000000000000444, 114.0000000000000000, 0.000000000000000000 ) ) ;
#8596=CARTESIAN_POINT ( 'NONE',  ( -1.915364268218909150, 110.6874999986344079, 1.915364268218909594 ) ) ;
#8615=CARTESIAN_POINT ( 'NONE',  ( 2.298097038856278918, 110.8750000000000000, -2.298097038856279806 ) ) ;
#8616=CARTESIAN_POINT ( 'NONE',  ( -1.121994411437819084, 113.8749999986344079, 2.708734124999999882 ) ) ;
#8627=FILL_AREA_STYLE_COLOUR ( '', #7580 ) ;
#8659=ORIENTED_EDGE ( 'NONE', *, *, #249, .F. ) ;
#8660=CARTESIAN_POINT ( 'NONE',  ( 1.658621287961228566E-16, 113.5624999986344079, 2.708734125000000326 ) ) ;
#8661=CARTESIAN_POINT ( 'NONE',  ( 3.249999999999999556, 111.8124999972688016, -1.346194077712561610 ) ) ;
#8671=CARTESIAN_POINT ( 'NONE',  ( 1.990051048614449116E-16, 110.2500000000000000, 3.250000000000000444 ) ) ;
#8673=CARTESIAN_POINT ( 'NONE',  ( -5.970153145843347347E-16, 113.6249999972688158, -3.250000000000000444 ) ) ;
#8691=CARTESIAN_POINT ( 'NONE',  ( -4.975863863883684959E-16, 111.0624999986344079, -2.708734125000000326 ) ) ;
#8704=LINE ( 'NONE', #4786, #11141 ) ;
#8709=ORIENTED_EDGE ( 'NONE', *, *, #2470, .F. ) ;
#8713=CARTESIAN_POINT ( 'NONE',  ( -3.250000000000001776, 111.4374999972688300, -1.346194077712558279 ) ) ;
#8718=CARTESIAN_POINT ( 'NONE',  ( 0.000000000000000000, 115.0000000000000000, 0.000000000000000000 ) ) ;
#8721=ORIENTED_EDGE ( 'NONE', *, *, #1152, .T. ) ;
#8722=LINE ( 'NONE', #2362, #7564 ) ;
#8723=CARTESIAN_POINT ( 'NONE',  ( 3.250000000000000444, 112.8749999972688158, 0.000000000000000000 ) ) ;
#8737=CARTESIAN_POINT ( 'NONE',  ( 1.121994411437819084, 113.7499999986344221, 2.708734124999999882 ) ) ;
#8752=ORIENTED_EDGE ( 'NONE', *, *, #10125, .T. ) ;
#8763=PRODUCT ( 'Central Drive Shaft Post', 'Central Drive Shaft Post', '', ( #1189 ) ) ;
#8782=CARTESIAN_POINT ( 'NONE',  ( -2.708734125000000326, 112.7499999986343937, 1.121994411437818862 ) ) ;
#8783=CARTESIAN_POINT ( 'NONE',  ( 1.346194077712559833, 113.6874999972688016, -3.250000000000000000 ) ) ;
#8793=CARTESIAN_POINT ( 'NONE',  ( -2.298097038856279806, 110.6250000000000000, -2.298097038856279362 ) ) ;
#8796=FACE_OUTER_BOUND ( 'NONE', #8849, .T. ) ;
#8798=CARTESIAN_POINT ( 'NONE',  ( 2.708734124999999882, 112.6249999986343937, 1.121994411437819084 ) ) ;
#8816=DIRECTION ( 'NONE',  ( -0.000000000000000000, 1.000000000000000000, -0.000000000000000000 ) ) ;
#8823=CARTESIAN_POINT ( 'NONE',  ( -1.915364268218909816, 111.9374999986344079, -1.915364268218909150 ) ) ;
#8824=ORIENTED_EDGE ( 'NONE', *, *, #1223, .F. ) ;
#8839=CARTESIAN_POINT ( 'NONE',  ( 1.658621287961228566E-16, 112.5624999986344079, 2.708734125000000326 ) ) ;
#8841=CARTESIAN_POINT ( 'NONE',  ( -3.250000000000000444, 114.3124999972688016, 1.346194077712559389 ) ) ;
#8842=ORIENTED_EDGE ( 'NONE', *, *, #9513, .T. ) ;
#8846=CIRCLE ( 'NONE', #6052, 3.250000000000000444 ) ;
#8849=EDGE_LOOP ( 'NONE', ( #8394, #1927, #60, #9862 ) ) ;
#8872=CARTESIAN_POINT ( 'NONE',  ( 1.915364268218909594, 110.4374999986344079, 1.915364268218909594 ) ) ;
#8878=EDGE_CURVE ( 'NONE', #9534, #1174, #8279, .T. ) ;
#8886=CARTESIAN_POINT ( 'NONE',  ( 1.915364268218908927, 114.1874999986344079, -1.915364268218909816 ) ) ;
#8893=ORIENTED_EDGE ( 'NONE', *, *, #4807, .T. ) ;
#8894=CARTESIAN_POINT ( 'NONE',  ( 0.000000000000000000, 110.0000000000000000, 3.250000000000000444 ) ) ;
#8905=DIRECTION ( 'NONE',  ( 0.000000000000000000, 0.000000000000000000, 1.000000000000000000 ) ) ;
#8914=ORIENTED_EDGE ( 'NONE', *, *, #11292, .F. ) ;
#8928=CARTESIAN_POINT ( 'NONE',  ( -2.298097038856279362, 112.2499999972688158, 2.298097038856279806 ) ) ;
#8943=CARTESIAN_POINT ( 'NONE',  ( 1.121994411437819528, 113.1249999986343937, -2.708734124999999882 ) ) ;
#8945=FACE_OUTER_BOUND ( 'NONE', #10973, .T. ) ;
#8955=DIRECTION ( 'NONE',  ( 0.000000000000000000, 0.000000000000000000, 1.000000000000000000 ) ) ;
#8958=CARTESIAN_POINT ( 'NONE',  ( 1.990051048614449116E-16, 113.2500000000000000, 3.250000000000000444 ) ) ;
#8984=FACE_OUTER_BOUND ( 'NONE', #1640, .T. ) ;
#9003=CARTESIAN_POINT ( 'NONE',  ( -1.121994411437820416, 113.9999999986343937, -2.708734124999999882 ) ) ;
#9005=ORIENTED_EDGE ( 'NONE', *, *, #9929, .F. ) ;
#9028=CARTESIAN_POINT ( 'NONE',  ( 0.000000000000000000, 165.0000000000000000, -9.999999999999998224 ) ) ;
#9035=CARTESIAN_POINT ( 'NONE',  ( 1.346194077712572934, 111.8124999999999858, -3.249999999999987121 ) ) ;
#9045=CARTESIAN_POINT ( 'NONE',  ( -8.000000000000000000, 165.0000000000000000, -5.999999999999998224 ) ) ;
#9066=CARTESIAN_POINT ( 'NONE',  ( 2.708734125000000326, 111.3124999986344079, 0.000000000000000000 ) ) ;
#9067=CARTESIAN_POINT ( 'NONE',  ( 1.658621287961228320E-16, 110.8124999986344079, 2.708734124999999882 ) ) ;
#9077=CARTESIAN_POINT ( 'NONE',  ( 0.000000000000000000, 153.0000000000000000, 0.000000000000000000 ) ) ;
#9085=DIRECTION ( 'NONE',  ( 1.000000000000000000, 0.000000000000000000, -0.000000000000000000 ) ) ;
#9086=ORIENTED_EDGE ( 'NONE', *, *, #1256, .T. ) ;
#9108=CARTESIAN_POINT ( 'NONE',  ( -2.708734125000000770, 112.8749999986344079, -1.121994411437818639 ) ) ;
#9157=( GEOMETRIC_REPRESENTATION_CONTEXT ( 3 ) GLOBAL_UNCERTAINTY_ASSIGNED_CONTEXT ( ( #1534 ) ) GLOBAL_UNIT_ASSIGNED_CONTEXT ( ( #1039, #4840, #6900 ) ) REPRESENTATION_CONTEXT ( 'NONE', 'WORKASPACE' ) );
#9163=ORIENTED_EDGE ( 'NONE', *, *, #5971, .F. ) ;
#9165=FACE_OUTER_BOUND ( 'NONE', #5214, .T. ) ;
#9172=CARTESIAN_POINT ( 'NONE',  ( -4.975863863883684959E-16, 114.0624999986344079, -2.708734125000000326 ) ) ;
#9174=CARTESIAN_POINT ( 'NONE',  ( 1.915364268218908705, 112.4374999986344079, -1.915364268218909594 ) ) ;
#9175=( BOUNDED_CURVE ( )  B_SPLINE_CURVE ( 2, ( #5666, #10452, #6776, #2784, #9571, #35, #3037, #11463, #12275 ),
 .UNSPECIFIED., .F., .F. ) 
 B_SPLINE_CURVE_WITH_KNOTS ( ( 3, 2, 2, 2, 3 ),
 ( 0.6875000000000005551, 0.7187500000000005551, 0.7500000000000006661, 0.7812500000000006661, 0.8125000000000006661 ),
 .UNSPECIFIED. ) 
 CURVE ( )  GEOMETRIC_REPRESENTATION_ITEM ( )  RATIONAL_B_SPLINE_CURVE ( ( 0.9999999999999986677, 0.9238795325112880708, 1.000000000000000000, 0.9238795325112867385, 1.000000000000000000, 0.9238795325112867385, 1.000000000000000000, 0.9238795325112850731, 1.000000000000001554 ) ) 
 REPRESENTATION_ITEM ( '' )  );
#9181=EDGE_CURVE ( 'NONE', #861, #9835, #11558, .T. ) ;
#9189=CARTESIAN_POINT ( 'NONE',  ( -1.346194077712560944, 112.6874999999999858, -3.249999999999999556 ) ) ;
#9236=CARTESIAN_POINT ( 'NONE',  ( 2.708734125000000326, 113.3749999986344079, 1.121994411437819084 ) ) ;
#9237=CARTESIAN_POINT ( 'NONE',  ( 3.250000000000000444, 114.8749999972688158, 0.000000000000000000 ) ) ;
#9246=VECTOR ( 'NONE', #1476, 1000.000000000000000 ) ;
#9253=ORIENTED_EDGE ( 'NONE', *, *, #4267, .F. ) ;
#9254=CARTESIAN_POINT ( 'NONE',  ( 2.298097038856278918, 111.8750000000000000, -2.298097038856279806 ) ) ;
#9267=LINE ( 'NONE', #2792, #3978 ) ;
#9287=CARTESIAN_POINT ( 'NONE',  ( -4.975863863883684959E-16, 114.3124999986344079, -2.708734124999999882 ) ) ;
#9293=DIRECTION ( 'NONE',  ( 0.000000000000000000, 0.000000000000000000, 1.000000000000000000 ) ) ;
#9298=CARTESIAN_POINT ( 'NONE',  ( -1.915364268218908927, 111.9374999986344079, 1.915364268218909150 ) ) ;
#9315=CARTESIAN_POINT ( 'NONE',  ( -2.298097038856279806, 113.6250000000000000, -2.298097038856279362 ) ) ;
#9343=CARTESIAN_POINT ( 'NONE',  ( -2.708734124999999882, 114.0624999986344079, 3.317242575922456639E-16 ) ) ;
#9359=CARTESIAN_POINT ( 'NONE',  ( -1.915364268218908927, 113.9374999986344079, 1.915364268218909150 ) ) ;
#9367=EDGE_CURVE ( 'NONE', #9534, #2576, #1754, .T. ) ;
#9393=AXIS2_PLACEMENT_3D ( 'NONE', #12041, #8905, #9085 ) ;
#9404=CARTESIAN_POINT ( 'NONE',  ( -1.915364268218909594, 112.1874999986344079, -1.915364268218908927 ) ) ;
#9407=FACE_OUTER_BOUND ( 'NONE', #10153, .T. ) ;
#9410=CARTESIAN_POINT ( 'NONE',  ( 0.000000000000000000, 153.0000000000000000, 0.000000000000000000 ) ) ;
#9419=CARTESIAN_POINT ( 'NONE',  ( 1.915364268218908705, 111.4374999986344079, -1.915364268218909594 ) ) ;
#9421=EDGE_CURVE ( 'NONE', #1550, #1153, #11504, .T. ) ;
#9428=ORIENTED_EDGE ( 'NONE', *, *, #249, .T. ) ;
#9430=DIRECTION ( 'NONE',  ( -0.000000000000000000, 1.000000000000000000, -0.000000000000000000 ) ) ;
#9451=VECTOR ( 'NONE', #11269, 1000.000000000000000 ) ;
#9471=CARTESIAN_POINT ( 'NONE',  ( -1.121994411437818862, 110.6249999986343937, 2.708734125000000326 ) ) ;
#9478=DIRECTION ( 'NONE',  ( -0.000000000000000000, 1.000000000000000000, -0.000000000000000000 ) ) ;
#9513=EDGE_CURVE ( 'NONE', #4699, #6802, #5806, .T. ) ;
#9520=CARTESIAN_POINT ( 'NONE',  ( -3.250000000000000444, 111.3749999972688158, 3.980102097228898231E-16 ) ) ;
#9528=CARTESIAN_POINT ( 'NONE',  ( 2.708734124999999882, 111.6249999986344079, 1.121994411437818862 ) ) ;
#9531=CARTESIAN_POINT ( 'NONE',  ( -1.346194077712560944, 113.5624999972688300, -3.249999999999999556 ) ) ;
#9534=VERTEX_POINT ( 'NONE', #1813 ) ;
#9538=CARTESIAN_POINT ( 'NONE',  ( 1.990051048614449116E-16, 110.2500000000000000, 3.250000000000000444 ) ) ;
#9540=ORIENTED_EDGE ( 'NONE', *, *, #11573, .F. ) ;
#9545=CARTESIAN_POINT ( 'NONE',  ( 2.708734124999999437, 114.4999999986344079, -1.121994411437820638 ) ) ;
#9546=CARTESIAN_POINT ( 'NONE',  ( 2.298097038856278918, 112.8750000000000000, -2.298097038856279806 ) ) ;
#9560=CARTESIAN_POINT ( 'NONE',  ( 2.979367062500000163, 114.1562499993171969, 0.000000000000000000 ) ) ;
#9562=CARTESIAN_POINT ( 'NONE',  ( 0.000000000000000000, 0.000000000000000000, 0.000000000000000000 ) ) ;
#9571=CARTESIAN_POINT ( 'NONE',  ( 3.250000000000000444, 113.0000000000000000, 0.000000000000000000 ) ) ;
#9577=EDGE_LOOP ( 'NONE', ( #8893, #4326, #4180, #9984 ) ) ;
#9592=EDGE_CURVE ( 'NONE', #11360, #7682, #10986, .T. ) ;
#9595=CARTESIAN_POINT ( 'NONE',  ( -4.975863863883684959E-16, 114.0624999986344079, -2.708734125000000326 ) ) ;
#9596=CARTESIAN_POINT ( 'NONE',  ( -3.250000000000000444, 113.3124999972688016, 1.346194077712559389 ) ) ;
#9605=DIRECTION ( 'NONE',  ( 0.000000000000000000, 0.000000000000000000, -1.000000000000000000 ) ) ;
#9609=CARTESIAN_POINT ( 'NONE',  ( -4.975863863883684959E-16, 114.3124999986344079, -2.708734124999999882 ) ) ;
#9638=VECTOR ( 'NONE', #5053, 1000.000000000000000 ) ;
#9646=ORIENTED_EDGE ( 'NONE', *, *, #124, .T. ) ;
#9653=CARTESIAN_POINT ( 'NONE',  ( -2.708734125000000326, 111.8124999986344079, 3.317242575922457132E-16 ) ) ;
#9654=CARTESIAN_POINT ( 'NONE',  ( -3.250000000000001776, 112.4374999972688300, -1.346194077712558723 ) ) ;
#9657=EDGE_CURVE ( 'NONE', #4316, #7882, #6663, .T. ) ;
#9671=CARTESIAN_POINT ( 'NONE',  ( -4.975863863883684959E-16, 113.3124999986344079, -2.708734124999999882 ) ) ;
#9683=CARTESIAN_POINT ( 'NONE',  ( 2.708734124999999882, 111.2499999986344079, -1.121994411437820416 ) ) ;
#9690=( NAMED_UNIT ( * ) PLANE_ANGLE_UNIT ( ) SI_UNIT ( $, .RADIAN. ) );
#9712=CARTESIAN_POINT ( 'NONE',  ( 2.708734125000000326, 112.3749999986344221, 1.121994411437818862 ) ) ;
#9713=CARTESIAN_POINT ( 'NONE',  ( -1.346194077712559389, 111.1874999972688016, 3.250000000000000444 ) ) ;
#9716=ORIENTED_EDGE ( 'NONE', *, *, #4410, .T. ) ;
#9728=DIRECTION ( 'NONE',  ( 0.000000000000000000, 0.000000000000000000, -1.000000000000000000 ) ) ;
#9729=CARTESIAN_POINT ( 'NONE',  ( 1.915364268218909150, 111.6874999986344079, 1.915364268218909150 ) ) ;
#9730=AXIS2_PLACEMENT_3D ( 'NONE', #2981, #2854, #3854 ) ;
#9747=ORIENTED_EDGE ( 'NONE', *, *, #3057, .F. ) ;
#9762=DIRECTION ( 'NONE',  ( 0.8660254037844410391, 0.4999999999999958367, -0.000000000000000000 ) ) ;
#9773=AXIS2_PLACEMENT_3D ( 'NONE', #1076, #7912, #10606 ) ;
#9778=CARTESIAN_POINT ( 'NONE',  ( -2.708734125000000770, 111.8749999986343937, -1.121994411437818639 ) ) ;
#9779=CARTESIAN_POINT ( 'NONE',  ( 1.346194077712559389, 114.0624999972688016, 3.250000000000000444 ) ) ;
#9788=VERTEX_POINT ( 'NONE', #7402 ) ;
#9789=FACE_OUTER_BOUND ( 'NONE', #618, .T. ) ;
#9812=PRESENTATION_STYLE_ASSIGNMENT (( #6027 ) ) ;
#9813=EDGE_CURVE ( 'NONE', #1550, #7936, #3592, .T. ) ;
#9821=CARTESIAN_POINT ( 'NONE',  ( 2.708734125000000326, 113.3124999986344079, 0.000000000000000000 ) ) ;
#9825=CIRCLE ( 'NONE', #8442, 9.999999999999998224 ) ;
#9826=EDGE_LOOP ( 'NONE', ( #42, #5094 ) ) ;
#9835=VERTEX_POINT ( 'NONE', #5343 ) ;
#9836=CARTESIAN_POINT ( 'NONE',  ( -1.121994411437820416, 112.9999999986343937, -2.708734124999999882 ) ) ;
#9862=ORIENTED_EDGE ( 'NONE', *, *, #5867, .T. ) ;
#9880=LINE ( 'NONE', #5909, #3496 ) ;
#9883=CARTESIAN_POINT ( 'NONE',  ( -2.708734125000000770, 113.8749999986343937, -1.121994411437818639 ) ) ;
#9884=VERTEX_POINT ( 'NONE', #917 ) ;
#9890=ORIENTED_EDGE ( 'NONE', *, *, #11848, .T. ) ;
#9901=CARTESIAN_POINT ( 'NONE',  ( -3.250000000000000444, 113.4375000000000000, 1.346194077712559167 ) ) ;
#9926=ORIENTED_EDGE ( 'NONE', *, *, #5822, .F. ) ;
#9927=CYLINDRICAL_SURFACE ( 'NONE', #850, 9.999999999999998224 ) ;
#9928=CARTESIAN_POINT ( 'NONE',  ( -3.250000000000000444, 112.3749999972688158, 3.980102097228898231E-16 ) ) ;
#9929=EDGE_CURVE ( 'NONE', #6802, #2738, #6709, .T. ) ;
#9940=CARTESIAN_POINT ( 'NONE',  ( 2.708734124999999882, 114.5624999986344079, 0.000000000000000000 ) ) ;
#9943=CARTESIAN_POINT ( 'NONE',  ( -2.708734125000000326, 111.8124999986344079, 3.317242575922457132E-16 ) ) ;
#9956=CARTESIAN_POINT ( 'NONE',  ( 3.250000000000000444, 113.9374999972688016, 1.346194077712559167 ) ) ;
#9962=CARTESIAN_POINT ( 'NONE',  ( -3.250000000000001776, 113.5625000000000000, -1.346194077712558279 ) ) ;
#9973=VERTEX_POINT ( 'NONE', #26 ) ;
#9984=ORIENTED_EDGE ( 'NONE', *, *, #4907, .T. ) ;
#9988=CARTESIAN_POINT ( 'NONE',  ( 2.298097038856279806, 111.1250000000000000, 2.298097038856279806 ) ) ;
#9994=CARTESIAN_POINT ( 'NONE',  ( 2.298097038856278918, 114.7499999972688158, -2.298097038856279806 ) ) ;
#10000=UNCERTAINTY_MEASURE_WITH_UNIT (LENGTH_MEASURE( 1.000000000000000082E-05 ), #7020, 'distance_accuracy_value', 'NONE');
#10010=CARTESIAN_POINT ( 'NONE',  ( 2.708734125000000326, 111.3749999986344221, 1.121994411437818862 ) ) ;
#10030=CARTESIAN_POINT ( 'NONE',  ( -2.298097038856279806, 114.4999999972688158, -2.298097038856279362 ) ) ;
#10040=CARTESIAN_POINT ( 'NONE',  ( -1.915364268218908927, 110.9374999986344079, 1.915364268218909150 ) ) ;
#10046=DIRECTION ( 'NONE',  ( -0.000000000000000000, 1.000000000000000000, -0.000000000000000000 ) ) ;
#10053=CARTESIAN_POINT ( 'NONE',  ( 1.658621287961228566E-16, 112.5624999986344079, 2.708734125000000326 ) ) ;
#10069=CARTESIAN_POINT ( 'NONE',  ( -1.346194077712560944, 111.6875000000000000, -3.249999999999999556 ) ) ;
#10071=PLANE ( 'NONE',  #3403 ) ;
#10086=CARTESIAN_POINT ( 'NONE',  ( -3.250000000000000444, 114.3124999972687874, 1.346194077712559167 ) ) ;
#10109=CARTESIAN_POINT ( 'NONE',  ( -2.708734125000000326, 113.8124999986344079, 3.317242575922457132E-16 ) ) ;
#10110=CARTESIAN_POINT ( 'NONE',  ( -1.915364268218908927, 110.9374999986344079, 1.915364268218909150 ) ) ;
#10124=EDGE_CURVE ( 'NONE', #12307, #2738, #3784, .T. ) ;
#10125=EDGE_CURVE ( 'NONE', #421, #4699, #2913, .T. ) ;
#10127=CARTESIAN_POINT ( 'NONE',  ( 3.250000000000000444, 112.0624999999999858, 1.346194077712559389 ) ) ;
#10139=DIRECTION ( 'NONE',  ( 0.000000000000000000, 0.000000000000000000, 1.000000000000000000 ) ) ;
#10149=DIRECTION ( 'NONE',  ( -0.000000000000000000, 1.000000000000000000, -0.000000000000000000 ) ) ;
#10153=EDGE_LOOP ( 'NONE', ( #7323, #9428, #90 ) ) ;
#10159=CARTESIAN_POINT ( 'NONE',  ( 1.346194077712557391, 111.0624999972687874, 3.250000000000002220 ) ) ;
#10160=STYLED_ITEM ( 'NONE', ( #3215 ), #7202 ) ;
#10175=CARTESIAN_POINT ( 'NONE',  ( 1.121994411437819528, 112.1249999986343937, -2.708734124999999882 ) ) ;
#10177=CARTESIAN_POINT ( 'NONE',  ( 1.121994411437818862, 113.7499999986343937, 2.708734124999999882 ) ) ;
#10192=CARTESIAN_POINT ( 'NONE',  ( -1.346194077712559389, 111.3125000000000142, 3.250000000000000444 ) ) ;
#10197=CARTESIAN_POINT ( 'NONE',  ( 1.346194077712544956, 113.0624999972688016, 3.250000000000015543 ) ) ;
#10212=CYLINDRICAL_SURFACE ( 'NONE', #5043, 3.250000000000000444 ) ;
#10224=CARTESIAN_POINT ( 'NONE',  ( 1.121994411437819084, 112.3749999986344221, -2.708734124999999437 ) ) ;
#10235=CARTESIAN_POINT ( 'NONE',  ( -1.346194077712542736, 112.6875000000000000, -3.250000000000017764 ) ) ;
#10237=ORIENTED_EDGE ( 'NONE', *, *, #4726, .F. ) ;
#10240=CARTESIAN_POINT ( 'NONE',  ( -5.970153145843347347E-16, 114.6249999972688158, -3.250000000000000444 ) ) ;
#10242=CIRCLE ( 'NONE', #3278, 3.250000000000000444 ) ;
#10256=CARTESIAN_POINT ( 'NONE',  ( -1.346194077712560944, 110.6875000000000000, -3.249999999999999556 ) ) ;
#10260=CARTESIAN_POINT ( 'NONE',  ( 3.250000000000000444, 112.8749999972688158, 0.000000000000000000 ) ) ;
#10266=ORIENTED_EDGE ( 'NONE', *, *, #8323, .F. ) ;
#10290=CARTESIAN_POINT ( 'NONE',  ( 1.915364268218909150, 112.6874999986344079, 1.915364268218909150 ) ) ;
#10301=CARTESIAN_POINT ( 'NONE',  ( 1.658621287961228320E-16, 110.8124999986344079, 2.708734124999999882 ) ) ;
#10306=CARTESIAN_POINT ( 'NONE',  ( -3.248205972160483255E-15, 151.7381927000421342, 0.000000000000000000 ) ) ;
#10309=VERTEX_POINT ( 'NONE', #8673 ) ;
#10316=CARTESIAN_POINT ( 'NONE',  ( -5.970153145843347347E-16, 111.7500000000000000, -3.250000000000000444 ) ) ;
#10328=VECTOR ( 'NONE', #9430, 1000.000000000000000 ) ;
#10346=CARTESIAN_POINT ( 'NONE',  ( -2.708734124999999882, 111.9999999986343937, 1.121994411437818862 ) ) ;
#10353=DIRECTION ( 'NONE',  ( -0.000000000000000000, 1.000000000000000000, -0.000000000000000000 ) ) ;
#10365=CARTESIAN_POINT ( 'NONE',  ( 1.121994411437818862, 110.7499999986343937, 2.708734124999999882 ) ) ;
#10367=ORIENTED_EDGE ( 'NONE', *, *, #4577, .F. ) ;
#10410=ORIENTED_EDGE ( 'NONE', *, *, #2470, .T. ) ;
#10411=CARTESIAN_POINT ( 'NONE',  ( 1.121994411437819084, 114.3749999986344221, -2.708734124999999437 ) ) ;
#10416=LINE ( 'NONE', #10603, #2983 ) ;
#10441=DIRECTION ( 'NONE',  ( -0.8660254037844408170, 0.4999999999999961697, -0.000000000000000000 ) ) ;
#10452=CARTESIAN_POINT ( 'NONE',  ( 1.346194077712578041, 112.8125000000000000, -3.249999999999981792 ) ) ;
#10461=ORIENTED_EDGE ( 'NONE', *, *, #2215, .T. ) ;
#10467=CARTESIAN_POINT ( 'NONE',  ( 2.979367062500000163, 110.1562499993171969, 0.000000000000000000 ) ) ;
#10480=CARTESIAN_POINT ( 'NONE',  ( -1.915364268218909594, 111.1874999986344079, -1.915364268218908927 ) ) ;
#10484=CARTESIAN_POINT ( 'NONE',  ( -8.000000000000000000, 165.0000000000000000, 5.999999999999998224 ) ) ;
#10492=CARTESIAN_POINT ( 'NONE',  ( -2.298097038856279806, 110.6250000000000000, -2.298097038856279362 ) ) ;
#10495=CARTESIAN_POINT ( 'NONE',  ( 2.708734124999999882, 114.5624999986344079, 0.000000000000000000 ) ) ;
#10530=DIRECTION ( 'NONE',  ( 0.000000000000000000, -1.000000000000000000, 0.000000000000000000 ) ) ;
#10534=CARTESIAN_POINT ( 'NONE',  ( 1.915364268218909594, 111.4374999986344079, 1.915364268218909594 ) ) ;
#10540=CARTESIAN_POINT ( 'NONE',  ( 3.250000000000000444, 110.8749999972688158, 0.000000000000000000 ) ) ;
#10553=CARTESIAN_POINT ( 'NONE',  ( -2.708734125000000326, 112.1249999986343937, -1.121994411437818195 ) ) ;
#10579=ORIENTED_EDGE ( 'NONE', *, *, #7001, .T. ) ;
#10580=CARTESIAN_POINT ( 'NONE',  ( -3.250000000000000444, 111.5000000000000000, 3.980102097228898231E-16 ) ) ;
#10581=DIRECTION ( 'NONE',  ( 0.000000000000000000, 0.000000000000000000, -1.000000000000000000 ) ) ;
#10592=CARTESIAN_POINT ( 'NONE',  ( -2.298097038856279362, 111.2499999972688158, 2.298097038856279806 ) ) ;
#10599=CARTESIAN_POINT ( 'NONE',  ( 2.708734125000000326, 114.3124999986344079, 0.000000000000000000 ) ) ;
#10600=CARTESIAN_POINT ( 'NONE',  ( -3.250000000000000444, 112.3124999972688016, 1.346194077712559389 ) ) ;
#10603=CARTESIAN_POINT ( 'NONE',  ( 0.000000000000000000, 165.0000000000000000, 2.099999999999993427 ) ) ;
#10606=DIRECTION ( 'NONE',  ( 0.000000000000000000, 0.000000000000000000, 1.000000000000000000 ) ) ;
#10616=CARTESIAN_POINT ( 'NONE',  ( -2.708734124999999882, 112.0624999986344079, 3.317242575922456639E-16 ) ) ;
#10625=CARTESIAN_POINT ( 'NONE',  ( -3.250000000000001776, 112.4374999972688300, -1.346194077712558279 ) ) ;
#10643=ORIENTED_EDGE ( 'NONE', *, *, #11654, .T. ) ;
#10660=CARTESIAN_POINT ( 'NONE',  ( 1.121994411437818862, 111.4999999986343937, 2.708734125000000326 ) ) ;
#10661=CARTESIAN_POINT ( 'NONE',  ( 1.990051048614449116E-16, 113.1249999972688158, 3.250000000000000444 ) ) ;
#10670=DIRECTION ( 'NONE',  ( -0.000000000000000000, 1.000000000000000000, -0.000000000000000000 ) ) ;
#10682=ORIENTED_EDGE ( 'NONE', *, *, #9657, .F. ) ;
#10687=CARTESIAN_POINT ( 'NONE',  ( 0.000000000000000000, 115.0000000000000000, 0.000000000000000000 ) ) ;
#10690=CARTESIAN_POINT ( 'NONE',  ( 2.708734125000000326, 110.3124999986344079, 0.000000000000000000 ) ) ;
#10700=CARTESIAN_POINT ( 'NONE',  ( 1.915364268218909594, 110.4374999986344079, 1.915364268218909594 ) ) ;
#10719=CARTESIAN_POINT ( 'NONE',  ( 2.708734125000000326, 111.3749999986344221, 1.121994411437818862 ) ) ;
#10720=CARTESIAN_POINT ( 'NONE',  ( -1.346194077712559389, 114.1874999972688016, 3.250000000000000444 ) ) ;
#10723=EDGE_CURVE ( 'NONE', #2576, #11144, #7903, .T. ) ;
#10728=FACE_OUTER_BOUND ( 'NONE', #5813, .T. ) ;
#10736=CARTESIAN_POINT ( 'NONE',  ( 1.915364268218908705, 112.4374999986344079, -1.915364268218909594 ) ) ;
#10767=CARTESIAN_POINT ( 'NONE',  ( 1.121994411437818862, 113.4999999986344079, 2.708734125000000326 ) ) ;
#10783=CARTESIAN_POINT ( 'NONE',  ( -2.708734125000000326, 113.8124999986344079, 3.317242575922457132E-16 ) ) ;
#10789=CYLINDRICAL_SURFACE ( 'NONE', #8465, 3.250000000000000444 ) ;
#10800=CARTESIAN_POINT ( 'NONE',  ( 2.298097038856279806, 111.9999999972688158, 2.298097038856279806 ) ) ;
#10825=CARTESIAN_POINT ( 'NONE',  ( 1.990051048614449116E-16, 110.2500000000000000, 3.250000000000000444 ) ) ;
#10833=EDGE_LOOP ( 'NONE', ( #9163, #4476, #403 ) ) ;
#10844=ADVANCED_FACE ( 'NONE', ( #2125, #11545 ), #5057, .F. ) ;
#10857=CARTESIAN_POINT ( 'NONE',  ( 2.708734124999999882, 110.5624999986344079, 0.000000000000000000 ) ) ;
#10875=CARTESIAN_POINT ( 'NONE',  ( -2.708734125000000326, 113.7499999986344221, 1.121994411437819084 ) ) ;
#10888=LINE ( 'NONE', #11708, #11843 ) ;
#10889=CARTESIAN_POINT ( 'NONE',  ( 1.121994411437819528, 112.1249999986343937, -2.708734124999999882 ) ) ;
#10931=CARTESIAN_POINT ( 'NONE',  ( -1.121994411437820194, 113.9999999986344079, -2.708734124999999882 ) ) ;
#10933=( BOUNDED_CURVE ( )  B_SPLINE_CURVE ( 2, ( #7215, #1545, #5290, #5708, #9067, #541, #3642, #3699, #2479, #4339, #11014, #1771, #11317, #8136, #4573, #7449, #2704, #2198, #9729, #7628, #14, #7868, #8552, #2956, #10616, #10553, #3018, #3829, #5946, #1210, #10736, #2143, #5016, #8798, #138, #4826, #11438, #6755, #3954, #6820, #11563, #6009, #265, #4077, #9671, #4952, #11506, #4013, #5890, #11629, #2021, #8737, #7814, #8616, #3078, #4759, #965, #2889, #11686, #3138, #6698, #5827, #6881, #2081, #10495 ),
 .UNSPECIFIED., .F., .F. ) 
 B_SPLINE_CURVE_WITH_KNOTS ( ( 3, 2, 2, 2, 2, 2, 2, 2, 2, 2, 2, 2, 2, 2, 2, 2, 2, 2, 2, 2, 2, 2, 2, 2, 2, 2, 2, 2, 2, 2, 2, 2, 3 ),
 ( 0.000000000000000000, 0.03125000000000000000, 0.06250000000000000000, 0.09375000000000000000, 0.1250000000000000000, 0.1562500000000000000, 0.1875000000000000000, 0.2187500000000000000, 0.2500000000000000000, 0.2812500000000000000, 0.3125000000000000000, 0.3437500000000000000, 0.3750000000000000000, 0.4062500000000000000, 0.4375000000000000000, 0.4687500000000000000, 0.5000000000000000000, 0.5312500000000000000, 0.5625000000000000000, 0.5937500000000000000, 0.6250000000000000000, 0.6562500000000000000, 0.6875000000000000000, 0.7187500000000000000, 0.7500000000000000000, 0.7812500000000000000, 0.8125000000000000000, 0.8437500000000000000, 0.8750000000000000000, 0.9062500000000000000, 0.9375000000000000000, 0.9687500000000000000, 1.000000000000000000 ),
 .UNSPECIFIED. ) 
 CURVE ( )  GEOMETRIC_REPRESENTATION_ITEM ( )  RATIONAL_B_SPLINE_CURVE ( ( 1.000000000000000000, 0.9238795325112867385, 1.000000000000000000, 0.9238795325112867385, 1.000000000000000000, 0.9238795325112867385, 1.000000000000000000, 0.9238795325112867385, 1.000000000000000000, 0.9238795325112867385, 1.000000000000000000, 0.9238795325112867385, 1.000000000000000000, 0.9238795325112867385, 1.000000000000000000, 0.9238795325112867385, 1.000000000000000000, 0.9238795325112867385, 1.000000000000000000, 0.9238795325112867385, 1.000000000000000000, 0.9238795325112867385, 1.000000000000000000, 0.9238795325112867385, 1.000000000000000000, 0.9238795325112867385, 1.000000000000000000, 0.9238795325112867385, 1.000000000000000000, 0.9238795325112867385, 1.000000000000000000, 0.9238795325112867385, 1.000000000000000000, 0.9238795325112867385, 1.000000000000000000, 0.9238795325112867385, 1.000000000000000000, 0.9238795325112867385, 1.000000000000000000, 0.9238795325112867385, 1.000000000000000000, 0.9238795325112867385, 1.000000000000000000, 0.9238795325112867385, 1.000000000000000000, 0.9238795325112867385, 1.000000000000000000, 0.9238795325112867385, 1.000000000000000000, 0.9238795325112867385, 1.000000000000000000, 0.9238795325112867385, 1.000000000000000000, 0.9238795325112867385, 1.000000000000000000, 0.9238795325112867385, 1.000000000000000000, 0.9238795325112867385, 1.000000000000000000, 0.9238795325112867385, 1.000000000000000000, 0.9238795325112867385, 1.000000000000000000, 0.9238795325112867385, 1.000000000000000000 ) ) 
 REPRESENTATION_ITEM ( '' )  );
#10942=CYLINDRICAL_SURFACE ( 'NONE', #4608, 3.250000000000000444 ) ;
#10947=CARTESIAN_POINT ( 'NONE',  ( -2.708734125000000770, 110.8749999986343937, -1.121994411437818639 ) ) ;
#10973=EDGE_LOOP ( 'NONE', ( #5055, #5697, #7860, #9716 ) ) ;
#10980=DIRECTION ( 'NONE',  ( 0.000000000000000000, 1.000000000000000000, 0.000000000000000000 ) ) ;
#10983=CARTESIAN_POINT ( 'NONE',  ( 1.658621287961228320E-16, 110.8124999986344079, 2.708734124999999882 ) ) ;
#10986=CIRCLE ( 'NONE', #2221, 9.999999999999998224 ) ;
#10989=CARTESIAN_POINT ( 'NONE',  ( 0.000000000000000000, 110.0000000000000000, 0.000000000000000000 ) ) ;
#10998=CARTESIAN_POINT ( 'NONE',  ( 1.915364268218909594, 111.4374999986344079, 1.915364268218909594 ) ) ;
#11007=CARTESIAN_POINT ( 'NONE',  ( 1.990051048614449116E-16, 112.2500000000000000, 3.250000000000000444 ) ) ;
#11012=CARTESIAN_POINT ( 'NONE',  ( -1.121994411437818862, 111.6249999986344079, 2.708734125000000326 ) ) ;
#11014=CARTESIAN_POINT ( 'NONE',  ( -1.915364268218909594, 111.1874999986344079, -1.915364268218908927 ) ) ;
#11026=ADVANCED_FACE ( 'NONE', ( #7104 ), #4350, .T. ) ;
#11043=AXIS2_PLACEMENT_3D ( 'NONE', #10989, #10046, #1520 ) ;
#11063=CARTESIAN_POINT ( 'NONE',  ( -2.708734125000000326, 111.8124999986344079, 3.317242575922457132E-16 ) ) ;
#11065=CARTESIAN_POINT ( 'NONE',  ( -4.975863863883684959E-16, 112.3124999986344079, -2.708734124999999882 ) ) ;
#11075=PLANE ( 'NONE',  #2029 ) ;
#11081=CYLINDRICAL_SURFACE ( 'NONE', #7358, 9.999999999999998224 ) ;
#11083=EDGE_CURVE ( 'NONE', #6351, #11360, #9267, .T. ) ;
#11091=CARTESIAN_POINT ( 'NONE',  ( 3.249999999999999556, 113.8124999972688016, -1.346194077712561166 ) ) ;
#11118=DIRECTION ( 'NONE',  ( 0.000000000000000000, 0.000000000000000000, 1.000000000000000000 ) ) ;
#11120=CARTESIAN_POINT ( 'NONE',  ( 2.298097038856278918, 110.8750000000000000, -2.298097038856279806 ) ) ;
#11125=CARTESIAN_POINT ( 'NONE',  ( 2.708734125000000326, 112.3124999986344079, 0.000000000000000000 ) ) ;
#11126=CARTESIAN_POINT ( 'NONE',  ( 2.708734124999999437, 113.4999999986344079, -1.121994411437820638 ) ) ;
#11139=CARTESIAN_POINT ( 'NONE',  ( 3.249999999999999556, 111.9374999999999858, -1.346194077712561610 ) ) ;
#11141=VECTOR ( 'NONE', #9762, 1000.000000000000114 ) ;
#11144=VERTEX_POINT ( 'NONE', #12032 ) ;
#11151=AXIS2_PLACEMENT_3D ( 'NONE', #6880, #11809, #6818 ) ;
#11157=CIRCLE ( 'NONE', #3779, 2.099999999999998312 ) ;
#11162=ORIENTED_EDGE ( 'NONE', *, *, #4103, .T. ) ;
#11174=CARTESIAN_POINT ( 'NONE',  ( -1.121994411437820194, 114.2499999986344079, -2.708734124999999437 ) ) ;
#11182=CARTESIAN_POINT ( 'NONE',  ( -1.346194077712573822, 112.3125000000000000, 3.249999999999985789 ) ) ;
#11190=CARTESIAN_POINT ( 'NONE',  ( -4.975863863883684959E-16, 111.3124999986344079, -2.708734124999999882 ) ) ;
#11204=EDGE_LOOP ( 'NONE', ( #2278, #1274, #4233, #8842 ) ) ;
#11205=CARTESIAN_POINT ( 'NONE',  ( 3.249999999999999556, 113.9374999999999858, -1.346194077712561610 ) ) ;
#11225=CARTESIAN_POINT ( 'NONE',  ( 3.980102097228898231E-16, 110.0000000000000000, -3.250000000000000444 ) ) ;
#11239=CARTESIAN_POINT ( 'NONE',  ( -4.975863863883684959E-16, 113.3124999986344079, -2.708734124999999882 ) ) ;
#11240=LINE ( 'NONE', #5568, #1814 ) ;
#11245=CARTESIAN_POINT ( 'NONE',  ( 1.224646799147353059E-15, 165.0000000000000000, 9.999999999999998224 ) ) ;
#11254=CARTESIAN_POINT ( 'NONE',  ( 2.708734124999999882, 112.6249999986343937, 1.121994411437818862 ) ) ;
#11269=DIRECTION ( 'NONE',  ( -0.000000000000000000, -1.000000000000000000, -0.000000000000000000 ) ) ;
#11275=ADVANCED_FACE ( 'NONE', ( #5792 ), #11402, .F. ) ;
#11276=CARTESIAN_POINT ( 'NONE',  ( 2.298097038856279806, 112.9999999972688158, 2.298097038856279806 ) ) ;
#11286=COLOUR_RGB ( '', 0.40784314, 0.44705882, 0.49803922) ;
#11291=EDGE_CURVE ( 'NONE', #5123, #5829, #11946, .T. ) ;
#11292=EDGE_CURVE ( 'NONE', #8492, #4699, #8704, .T. ) ;
#11295=CARTESIAN_POINT ( 'NONE',  ( 0.000000000000000000, 110.0000000000000000, 0.000000000000000000 ) ) ;
#11299=ORIENTED_EDGE ( 'NONE', *, *, #9421, .F. ) ;
#11304=CARTESIAN_POINT ( 'NONE',  ( 1.121994411437818862, 110.4999999986344079, 2.708734125000000326 ) ) ;
#11316=CARTESIAN_POINT ( 'NONE',  ( 1.346194077712559833, 114.6874999972688158, -3.250000000000000000 ) ) ;
#11317=CARTESIAN_POINT ( 'NONE',  ( -4.975863863883684959E-16, 111.3124999986344079, -2.708734124999999882 ) ) ;
#11341=ADVANCED_FACE ( 'NONE', ( #7592 ), #5074, .F. ) ;
#11356=ADVANCED_FACE ( 'NONE', ( #7627 ), #11081, .T. ) ;
#11360=VERTEX_POINT ( 'NONE', #325 ) ;
#11361=CARTESIAN_POINT ( 'NONE',  ( -2.708734124999999882, 113.9999999986343937, 1.121994411437818862 ) ) ;
#11362=DIRECTION ( 'NONE',  ( 0.000000000000000000, -1.000000000000000000, 0.000000000000000000 ) ) ;
#11367=( BOUNDED_CURVE ( )  B_SPLINE_CURVE ( 2, ( #5678, #5923, #10592, #239, #9520, #8713, #5740, #7543, #1933 ),
 .UNSPECIFIED., .F., .T. ) 
 B_SPLINE_CURVE_WITH_KNOTS ( ( 3, 2, 2, 2, 3 ),
 ( 0.06250000000000005551, 0.09375000000000008327, 0.1250000000000001110, 0.1562500000000001388, 0.1875000000000001665 ),
 .UNSPECIFIED. ) 
 CURVE ( )  GEOMETRIC_REPRESENTATION_ITEM ( )  RATIONAL_B_SPLINE_CURVE ( ( 0.9999999999999998890, 0.9238795325112868495, 1.000000000000000000, 0.9238795325112867385, 1.000000000000000000, 0.9238795325112867385, 1.000000000000000000, 0.9238795325112862944, 1.000000000000000444 ) ) 
 REPRESENTATION_ITEM ( '' )  );
#11383=FACE_OUTER_BOUND ( 'NONE', #3233, .T. ) ;
#11388=VECTOR ( 'NONE', #665, 1000.000000000000000 ) ;
#11402=CYLINDRICAL_SURFACE ( 'NONE', #9730, 2.099999999999993427 ) ;
#11405=DIRECTION ( 'NONE',  ( -0.8660254037844410391, -0.4999999999999958367, 0.000000000000000000 ) ) ;
#11409=DIRECTION ( 'NONE',  ( -1.734723475976805517E-15, 1.000000000000000000, -0.000000000000000000 ) ) ;
#11420=ORIENTED_EDGE ( 'NONE', *, *, #7466, .T. ) ;
#11421=CARTESIAN_POINT ( 'NONE',  ( 1.658621287961228320E-16, 111.8124999986344079, 2.708734124999999882 ) ) ;
#11422=CARTESIAN_POINT ( 'NONE',  ( -2.298097038856279806, 113.4999999972688158, -2.298097038856279362 ) ) ;
#11433=ADVANCED_FACE ( 'NONE', ( #8796 ), #7748, .T. ) ;
#11437=CARTESIAN_POINT ( 'NONE',  ( -3.250000000000000444, 110.5000000000000000, 3.980102097228898231E-16 ) ) ;
#11438=CARTESIAN_POINT ( 'NONE',  ( 1.658621287961228320E-16, 112.8124999986344079, 2.708734124999999882 ) ) ;
#11443=( BOUNDED_CURVE ( )  B_SPLINE_CURVE ( 2, ( #8958, #5124, #7106, #9901, #4297, #9962, #3303, #5180, #8151 ),
 .UNSPECIFIED., .F., .F. ) 
 B_SPLINE_CURVE_WITH_KNOTS ( ( 3, 2, 2, 2, 3 ),
 ( 0.8125000000000006661, 0.8437500000000006661, 0.8750000000000006661, 0.9062500000000007772, 0.9375000000000007772 ),
 .UNSPECIFIED. ) 
 CURVE ( )  GEOMETRIC_REPRESENTATION_ITEM ( )  RATIONAL_B_SPLINE_CURVE ( ( 0.9999999999999983347, 0.9238795325112884038, 1.000000000000000000, 0.9238795325112867385, 1.000000000000000000, 0.9238795325112867385, 1.000000000000000000, 0.9238795325112848511, 1.000000000000001998 ) ) 
 REPRESENTATION_ITEM ( '' )  );
#11455=AXIS2_PLACEMENT_3D ( 'NONE', #6239, #3372, #5306 ) ;
#11463=CARTESIAN_POINT ( 'NONE',  ( 1.346194077712537629, 113.1875000000000284, 3.250000000000022649 ) ) ;
#11465=ORIENTED_EDGE ( 'NONE', *, *, #8493, .F. ) ;
#11472=ADVANCED_FACE ( 'NONE', ( #11685 ), #1149, .T. ) ;
#11488=CARTESIAN_POINT ( 'NONE',  ( -1.121994411437820416, 113.9999999986343937, -2.708734124999999882 ) ) ;
#11503=CARTESIAN_POINT ( 'NONE',  ( -2.298097038856279362, 111.3750000000000000, 2.298097038856279806 ) ) ;
#11504=CIRCLE ( 'NONE', #6711, 9.999999999999998224 ) ;
#11506=CARTESIAN_POINT ( 'NONE',  ( 1.915364268218908705, 113.4374999986344079, -1.915364268218909594 ) ) ;
#11524=DIRECTION ( 'NONE',  ( 0.000000000000000000, 0.000000000000000000, 1.000000000000000000 ) ) ;
#11545=FACE_OUTER_BOUND ( 'NONE', #6722, .T. ) ;
#11547=CARTESIAN_POINT ( 'NONE',  ( 2.708734124999999882, 114.2499999986344079, -1.121994411437820638 ) ) ;
#11548=CARTESIAN_POINT ( 'NONE',  ( -2.298097038856279362, 112.2499999972688158, 2.298097038856279806 ) ) ;
#11557=CARTESIAN_POINT ( 'NONE',  ( -5.970153145843347347E-16, 110.7500000000000000, -3.250000000000000444 ) ) ;
#11558=LINE ( 'NONE', #5886, #337 ) ;
#11563=CARTESIAN_POINT ( 'NONE',  ( -2.708734124999999882, 113.0624999986344079, 3.317242575922456639E-16 ) ) ;
#11573=EDGE_CURVE ( 'NONE', #12241, #1921, #11745, .T. ) ;
#11591=CARTESIAN_POINT ( 'NONE',  ( -1.346194077712548287, 111.6875000000000000, -3.250000000000012434 ) ) ;
#11595=CARTESIAN_POINT ( 'NONE',  ( -3.250000000000000444, 113.3749999972688158, 3.980102097228898231E-16 ) ) ;
#11613=CARTESIAN_POINT ( 'NONE',  ( 3.250000000000000444, 111.9374999972688016, 1.346194077712559389 ) ) ;
#11627=DIRECTION ( 'NONE',  ( 0.000000000000000000, 0.000000000000000000, -1.000000000000000000 ) ) ;
#11629=CARTESIAN_POINT ( 'NONE',  ( 2.708734124999999882, 113.6249999986344079, 1.121994411437819084 ) ) ;
#11642=ADVANCED_FACE ( 'NONE', ( #7121 ), #8400, .F. ) ;
#11645=CARTESIAN_POINT ( 'NONE',  ( 0.000000000000000000, 110.0000000000000000, 0.000000000000000000 ) ) ;
#11654=EDGE_CURVE ( 'NONE', #4316, #9884, #8722, .T. ) ;
#11669=CARTESIAN_POINT ( 'NONE',  ( 2.708734124999999882, 112.2499999986344079, -1.121994411437820638 ) ) ;
#11670=CARTESIAN_POINT ( 'NONE',  ( -3.250000000000001776, 114.4374999972688158, -1.346194077712558723 ) ) ;
#11685=FACE_OUTER_BOUND ( 'NONE', #11204, .T. ) ;
#11686=CARTESIAN_POINT ( 'NONE',  ( -1.915364268218909594, 114.1874999986344079, -1.915364268218908927 ) ) ;
#11703=SURFACE_STYLE_FILL_AREA ( #2103 ) ;
#11708=CARTESIAN_POINT ( 'NONE',  ( 0.000000000000000000, 110.0000000000000000, 3.250000000000000444 ) ) ;
#11709=CARTESIAN_POINT ( 'NONE',  ( -4.975863863883684959E-16, 112.0624999986344079, -2.708734125000000326 ) ) ;
#11720=EDGE_CURVE ( 'NONE', #2552, #12150, #11443, .T. ) ;
#11726=CARTESIAN_POINT ( 'NONE',  ( 1.915364268218909594, 113.4374999986344079, 1.915364268218909594 ) ) ;
#11745=( BOUNDED_CURVE ( )  B_SPLINE_CURVE ( 2, ( #1575, #9035, #637, #7183, #6251, #5377, #509, #5317, #7312 ),
 .UNSPECIFIED., .F., .T. ) 
 B_SPLINE_CURVE_WITH_KNOTS ( ( 3, 2, 2, 2, 3 ),
 ( 0.4375000000000003886, 0.4687500000000003886, 0.5000000000000004441, 0.5312500000000004441, 0.5625000000000004441 ),
 .UNSPECIFIED. ) 
 CURVE ( )  GEOMETRIC_REPRESENTATION_ITEM ( )  RATIONAL_B_SPLINE_CURVE ( ( 0.9999999999999990008, 0.9238795325112877377, 1.000000000000000000, 0.9238795325112867385, 1.000000000000000000, 0.9238795325112867385, 1.000000000000000000, 0.9238795325112856283, 1.000000000000001110 ) ) 
 REPRESENTATION_ITEM ( '' )  );
#11755=ORIENTED_EDGE ( 'NONE', *, *, #10125, .F. ) ;
#11756=FACE_OUTER_BOUND ( 'NONE', #7892, .T. ) ;
#11760=CARTESIAN_POINT ( 'NONE',  ( 1.658621287961228566E-16, 110.5624999986344079, 2.708734125000000326 ) ) ;
#11770=( BOUNDED_CURVE ( )  B_SPLINE_CURVE ( 2, ( #3297, #4412, #8205, #11091, #6162, #9956, #489, #2546, #11787 ),
 .UNSPECIFIED., .F., .F. ) 
 B_SPLINE_CURVE_WITH_KNOTS ( ( 3, 2, 2, 2, 3 ),
 ( 0.6875000000000005551, 0.7187500000000005551, 0.7500000000000006661, 0.7812500000000006661, 0.8125000000000006661 ),
 .UNSPECIFIED. ) 
 CURVE ( )  GEOMETRIC_REPRESENTATION_ITEM ( )  RATIONAL_B_SPLINE_CURVE ( ( 0.9999999999999986677, 0.9238795325112880708, 1.000000000000000000, 0.9238795325112867385, 1.000000000000000000, 0.9238795325112867385, 1.000000000000000000, 0.9238795325112850731, 1.000000000000001554 ) ) 
 REPRESENTATION_ITEM ( '' )  );
#11778=CARTESIAN_POINT ( 'NONE',  ( 2.298097038856279806, 110.1250000000000000, 2.298097038856279806 ) ) ;
#11787=CARTESIAN_POINT ( 'NONE',  ( 1.990051048614449116E-16, 114.1249999972688158, 3.250000000000000444 ) ) ;
#11809=DIRECTION ( 'NONE',  ( -0.000000000000000000, 1.000000000000000000, -0.000000000000000000 ) ) ;
#11825=CARTESIAN_POINT ( 'NONE',  ( -2.708734125000000326, 111.7499999986343795, 1.121994411437819084 ) ) ;
#11838=CARTESIAN_POINT ( 'NONE',  ( 1.915364268218908927, 111.1874999986344079, -1.915364268218909816 ) ) ;
#11843=VECTOR ( 'NONE', #6908, 1000.000000000000000 ) ;
#11848=EDGE_CURVE ( 'NONE', #2576, #2418, #8399, .T. ) ;
#11851=CARTESIAN_POINT ( 'NONE',  ( -5.970153145843347347E-16, 110.7500000000000000, -3.250000000000000444 ) ) ;
#11860=CARTESIAN_POINT ( 'NONE',  ( -3.250000000000001776, 114.4374999972688158, -1.346194077712558279 ) ) ;
#11872=AXIS2_PLACEMENT_3D ( 'NONE', #4067, #10670, #6812 ) ;
#11884=CARTESIAN_POINT ( 'NONE',  ( -1.915364268218909150, 111.6874999986344079, 1.915364268218909594 ) ) ;
#11896=( BOUNDED_CURVE ( )  B_SPLINE_CURVE ( 2, ( #7502, #1826, #1948, #12305, #9538 ),
 .UNSPECIFIED., .F., .F. ) 
 B_SPLINE_CURVE_WITH_KNOTS ( ( 3, 2, 3 ),
 ( 0.000000000000000000, 0.03125000000000002776, 0.06250000000000005551 ),
 .UNSPECIFIED. ) 
 CURVE ( )  GEOMETRIC_REPRESENTATION_ITEM ( )  RATIONAL_B_SPLINE_CURVE ( ( 1.000000000000000000, 0.9238795325112867385, 1.000000000000000000, 0.9238795325112866275, 1.000000000000000222 ) ) 
 REPRESENTATION_ITEM ( '' )  );
#11901=CARTESIAN_POINT ( 'NONE',  ( -2.708734125000000326, 112.8124999986344079, 3.317242575922457132E-16 ) ) ;
#11923=DIRECTION ( 'NONE',  ( 0.000000000000000000, 0.000000000000000000, 1.000000000000000000 ) ) ;
#11941=CARTESIAN_POINT ( 'NONE',  ( 1.121994411437819084, 112.4999999986343937, 2.708734125000000326 ) ) ;
#11944=ORIENTED_EDGE ( 'NONE', *, *, #9367, .F. ) ;
#11946=CIRCLE ( 'NONE', #6568, 3.250000000000000444 ) ;
#11956=CARTESIAN_POINT ( 'NONE',  ( 3.250000000000000444, 110.0624999999999858, 1.346194077712559389 ) ) ;
#11976=EDGE_CURVE ( 'NONE', #7882, #10309, #5395, .T. ) ;
#11982=CARTESIAN_POINT ( 'NONE',  ( -5.970153145843347347E-16, 114.6249999972688158, -3.250000000000000444 ) ) ;
#11989=CARTESIAN_POINT ( 'NONE',  ( 3.980102097228898231E-16, 115.0000000000000000, -3.250000000000000444 ) ) ;
#12005=CARTESIAN_POINT ( 'NONE',  ( 1.658621287961228566E-16, 113.5624999986344079, 2.708734125000000326 ) ) ;
#12018=CARTESIAN_POINT ( 'NONE',  ( -5.970153145843347347E-16, 111.6249999972688158, -3.250000000000000444 ) ) ;
#12019=CARTESIAN_POINT ( 'NONE',  ( 1.990051048614449116E-16, 111.2500000000000000, 3.250000000000000444 ) ) ;
#12020=VECTOR ( 'NONE', #8570, 1000.000000000000000 ) ;
#12032=CARTESIAN_POINT ( 'NONE',  ( 1.990051048614449116E-16, 111.1249999972688158, 3.250000000000000444 ) ) ;
#12041=CARTESIAN_POINT ( 'NONE',  ( 2.979367062500000163, 110.1562499993171969, 0.000000000000000000 ) ) ;
#12058=CYLINDRICAL_SURFACE ( 'NONE', #1497, 3.250000000000000444 ) ;
#12066=CARTESIAN_POINT ( 'NONE',  ( -2.708734125000000326, 112.8124999986344079, 3.317242575922457132E-16 ) ) ;
#12068=CARTESIAN_POINT ( 'NONE',  ( -1.915364268218909594, 113.1874999986344079, -1.915364268218908927 ) ) ;
#12085=CARTESIAN_POINT ( 'NONE',  ( 3.250000000000000444, 111.8749999972688158, 0.000000000000000000 ) ) ;
#12087=CARTESIAN_POINT ( 'NONE',  ( -5.970153145843347347E-16, 111.7500000000000000, -3.250000000000000444 ) ) ;
#12096=CARTESIAN_POINT ( 'NONE',  ( 3.980102097228898231E-16, 110.0000000000000000, -3.250000000000000444 ) ) ;
#12101=ADVANCED_FACE ( 'NONE', ( #418 ), #480, .T. ) ;
#12114=CARTESIAN_POINT ( 'NONE',  ( -1.915364268218908927, 113.9374999986344079, 1.915364268218909150 ) ) ;
#12130=CARTESIAN_POINT ( 'NONE',  ( 2.708734124999999882, 112.5624999986344079, 0.000000000000000000 ) ) ;
#12144=CARTESIAN_POINT ( 'NONE',  ( -5.970153145843347347E-16, 113.7500000000000000, -3.250000000000000444 ) ) ;
#12145=ADVANCED_FACE ( 'NONE', ( #5167, #8945 ), #10071, .T. ) ;
#12147=AXIS2_PLACEMENT_3D ( 'NONE', #4416, #5122, #6048 ) ;
#12150=VERTEX_POINT ( 'NONE', #6282 ) ;
#12174=DIRECTION ( 'NONE',  ( 0.000000000000000000, 1.000000000000000000, 0.000000000000000000 ) ) ;
#12177=CARTESIAN_POINT ( 'NONE',  ( -2.708734124999999882, 110.9999999986343937, 1.121994411437818862 ) ) ;
#12184=CARTESIAN_POINT ( 'NONE',  ( 1.990051048614449116E-16, 113.2500000000000000, 3.250000000000000444 ) ) ;
#12193=CARTESIAN_POINT ( 'NONE',  ( 1.658621287961228320E-16, 113.8124999986344079, 2.708734124999999882 ) ) ;
#12221=VECTOR ( 'NONE', #5231, 1000.000000000000227 ) ;
#12226=DIRECTION ( 'NONE',  ( 0.000000000000000000, 0.000000000000000000, 1.000000000000000000 ) ) ;
#12239=CARTESIAN_POINT ( 'NONE',  ( 2.708734125000000326, 110.3749999986344221, 1.121994411437818862 ) ) ;
#12241=VERTEX_POINT ( 'NONE', #10316 ) ;
#12252=CARTESIAN_POINT ( 'NONE',  ( 3.249999999999999556, 114.8124999972688016, -1.346194077712561610 ) ) ;
#12275=CARTESIAN_POINT ( 'NONE',  ( 1.990051048614449116E-16, 113.2500000000000000, 3.250000000000000444 ) ) ;
#12284=ORIENTED_EDGE ( 'NONE', *, *, #6662, .F. ) ;
#12295=DIRECTION ( 'NONE',  ( 0.000000000000000000, 0.000000000000000000, 1.000000000000000000 ) ) ;
#12298=CARTESIAN_POINT ( 'NONE',  ( -1.121994411437818862, 111.8749999986343937, 2.708734124999999882 ) ) ;
#12305=CARTESIAN_POINT ( 'NONE',  ( 1.346194077712557391, 110.1875000000000000, 3.250000000000002220 ) ) ;
#12307=VERTEX_POINT ( 'NONE', #2600 ) ;
#12310=CARTESIAN_POINT ( 'NONE',  ( 2.298097038856278918, 114.7499999972688158, -2.298097038856279806 ) ) ;
#12314=( BOUNDED_CURVE ( )  B_SPLINE_CURVE ( 2, ( #2109, #8575, #101, #7653, #10580, #5669, #7773, #11591, #7833 ),
 .UNSPECIFIED., .F., .F. ) 
 B_SPLINE_CURVE_WITH_KNOTS ( ( 3, 2, 2, 2, 3 ),
 ( 0.3125000000000002776, 0.3437500000000003331, 0.3750000000000003331, 0.4062500000000003331, 0.4375000000000003886 ),
 .UNSPECIFIED. ) 
 CURVE ( )  GEOMETRIC_REPRESENTATION_ITEM ( )  RATIONAL_B_SPLINE_CURVE ( ( 0.9999999999999993339, 0.9238795325112874046, 1.000000000000000000, 0.9238795325112867385, 1.000000000000000000, 0.9238795325112867385, 1.000000000000000000, 0.9238795325112857393, 1.000000000000000888 ) ) 
 REPRESENTATION_ITEM ( '' )  );
#12315=ORIENTED_EDGE ( 'NONE', *, *, #5382, .F. ) ;
#12334=LINE ( 'NONE', #3723, #707 ) ;
ENDSEC;
END-ISO-10303-21;
